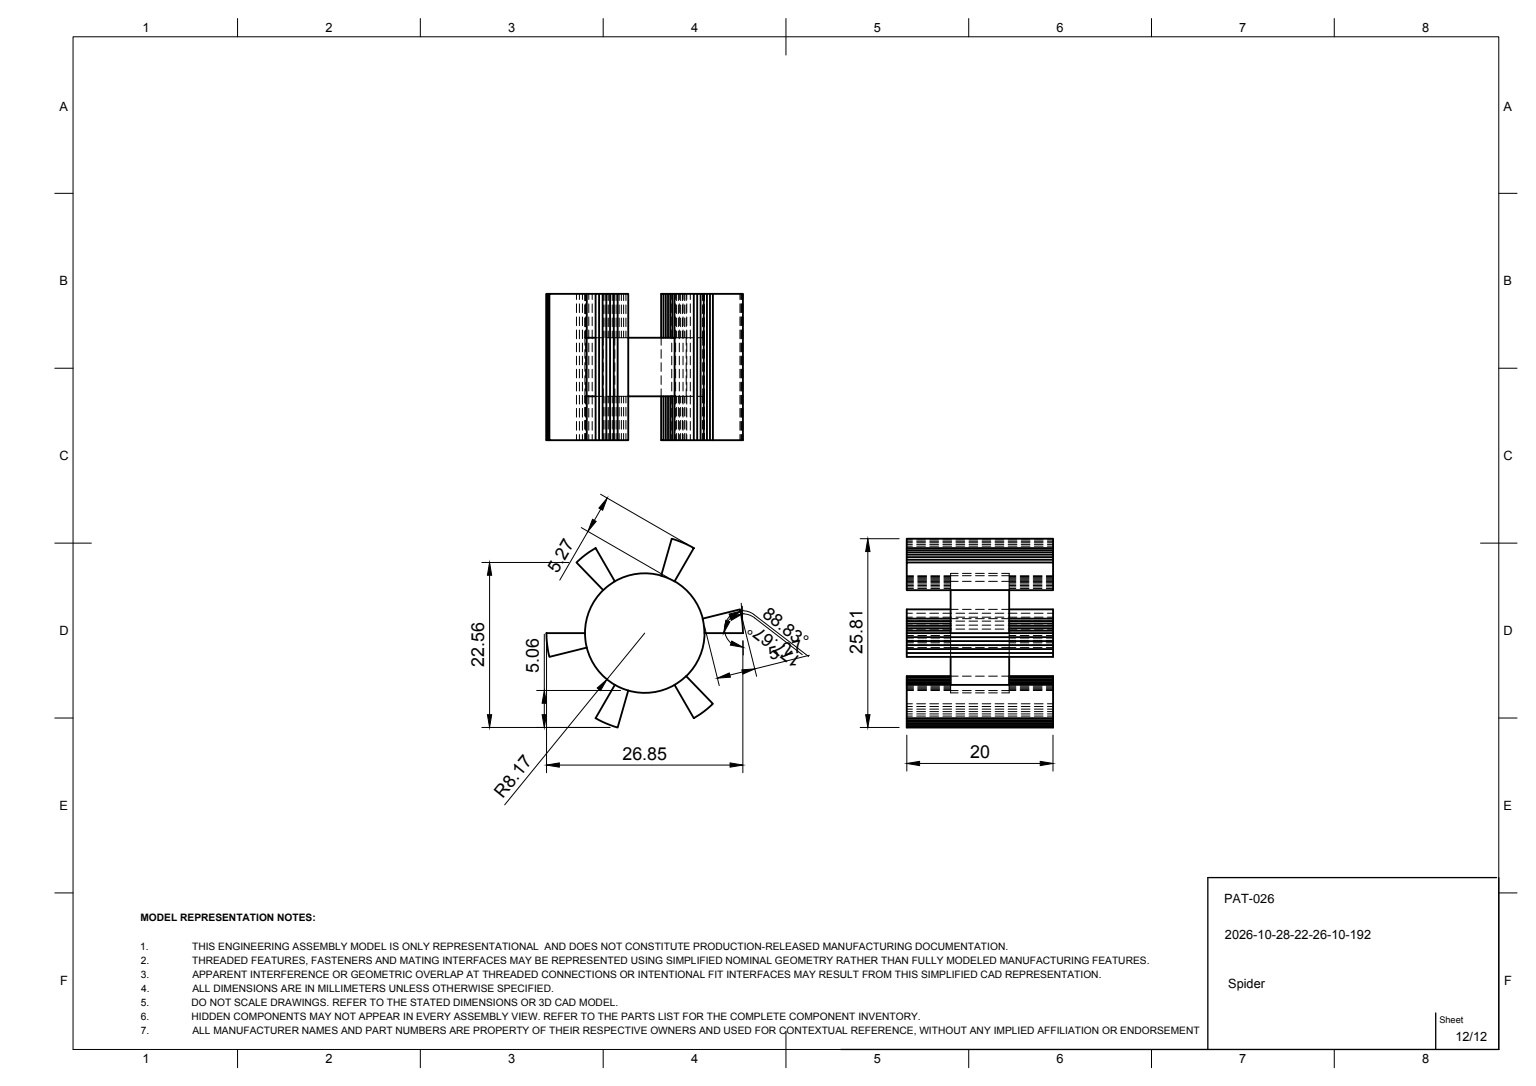
ISO-10303-21;
HEADER;
/* Generated by software containing ST-Developer
 * from STEP Tools, Inc. (www.steptools.com) 
 */

FILE_DESCRIPTION(
/* description */ ('PAT-026'),
/* implementation_level */ '2;1');

FILE_NAME(
/* name */ 'Spider.step',
/* time_stamp */ '2026-10-28T22:25:58-07:00',
/* author */ (''),
/* organization */ (''),
/* preprocessor_version */ 'ST-DEVELOPER v20.2',
/* originating_system */ 'Autodesk Translation Framework v15.17.0.0',
/* authorisation */ '');

FILE_SCHEMA (('AUTOMOTIVE_DESIGN { 1 0 10303 214 3 1 1 }'));
ENDSEC;

DATA;
#10=MECHANICAL_DESIGN_GEOMETRIC_PRESENTATION_REPRESENTATION('',(#150),#12343);
#128=SHAPE_REPRESENTATION_RELATIONSHIP('SRR','None',#12406,#139);
#139=ADVANCED_BREP_SHAPE_REPRESENTATION('',(#159),#12341);
#150=STYLED_ITEM('',(#12526),#159);
#159=MANIFOLD_SOLID_BREP('Body1',#7358);
#410=PLANE('',#7854);
#411=PLANE('',#7873);
#412=PLANE('',#7874);
#413=PLANE('',#7875);
#414=PLANE('',#7876);
#415=PLANE('',#7877);
#416=PLANE('',#7878);
#417=PLANE('',#7879);
#418=PLANE('',#7880);
#419=PLANE('',#7881);
#420=PLANE('',#7882);
#421=PLANE('',#7883);
#422=PLANE('',#7884);
#423=PLANE('',#7885);
#424=PLANE('',#7886);
#425=PLANE('',#7887);
#426=PLANE('',#7888);
#427=PLANE('',#7889);
#428=PLANE('',#7890);
#429=PLANE('',#7891);
#430=PLANE('',#7892);
#431=PLANE('',#7893);
#432=PLANE('',#7894);
#433=PLANE('',#7895);
#434=PLANE('',#7896);
#435=PLANE('',#7897);
#436=PLANE('',#7898);
#437=PLANE('',#7899);
#438=PLANE('',#7900);
#439=PLANE('',#7901);
#440=PLANE('',#7902);
#441=PLANE('',#7903);
#442=PLANE('',#7904);
#443=PLANE('',#7905);
#444=PLANE('',#7906);
#445=PLANE('',#7907);
#446=PLANE('',#7908);
#447=PLANE('',#7909);
#448=PLANE('',#7910);
#449=PLANE('',#7911);
#450=PLANE('',#7912);
#451=PLANE('',#7913);
#452=PLANE('',#7914);
#453=PLANE('',#7915);
#454=PLANE('',#7916);
#455=PLANE('',#7917);
#456=PLANE('',#7918);
#457=PLANE('',#7919);
#458=PLANE('',#7920);
#459=PLANE('',#7921);
#460=PLANE('',#7922);
#461=PLANE('',#7923);
#462=PLANE('',#7924);
#463=PLANE('',#7925);
#464=PLANE('',#7926);
#465=PLANE('',#7927);
#466=PLANE('',#7928);
#467=PLANE('',#7929);
#468=PLANE('',#7930);
#469=PLANE('',#7931);
#470=PLANE('',#7932);
#471=PLANE('',#7933);
#472=PLANE('',#7934);
#473=PLANE('',#7935);
#474=PLANE('',#7936);
#475=PLANE('',#7937);
#476=PLANE('',#7938);
#477=PLANE('',#7939);
#478=PLANE('',#7940);
#479=PLANE('',#7941);
#480=PLANE('',#7942);
#481=PLANE('',#7943);
#482=PLANE('',#7944);
#483=PLANE('',#7945);
#484=PLANE('',#7946);
#485=PLANE('',#7947);
#486=PLANE('',#7948);
#487=PLANE('',#7949);
#488=PLANE('',#7950);
#489=PLANE('',#7951);
#490=PLANE('',#7952);
#491=PLANE('',#7953);
#492=PLANE('',#7954);
#493=PLANE('',#7955);
#494=PLANE('',#7956);
#495=PLANE('',#7957);
#496=PLANE('',#7958);
#497=PLANE('',#7959);
#498=PLANE('',#7960);
#499=PLANE('',#7961);
#500=PLANE('',#7962);
#501=PLANE('',#7963);
#502=PLANE('',#7964);
#503=PLANE('',#7965);
#504=PLANE('',#7966);
#505=PLANE('',#7967);
#506=PLANE('',#7968);
#507=PLANE('',#7969);
#508=PLANE('',#7970);
#509=PLANE('',#7971);
#510=PLANE('',#7972);
#511=PLANE('',#7973);
#512=PLANE('',#7974);
#513=PLANE('',#7975);
#514=PLANE('',#7976);
#515=PLANE('',#7977);
#516=PLANE('',#7978);
#517=PLANE('',#7979);
#518=PLANE('',#7980);
#519=PLANE('',#7981);
#520=PLANE('',#7982);
#521=PLANE('',#7983);
#522=PLANE('',#7984);
#523=PLANE('',#7985);
#524=PLANE('',#7986);
#525=PLANE('',#7987);
#526=PLANE('',#7988);
#527=PLANE('',#7989);
#528=PLANE('',#7990);
#529=PLANE('',#7991);
#530=PLANE('',#7992);
#531=PLANE('',#7993);
#532=PLANE('',#7994);
#533=PLANE('',#7995);
#534=PLANE('',#7996);
#535=PLANE('',#7997);
#536=PLANE('',#7998);
#537=PLANE('',#7999);
#538=PLANE('',#8000);
#539=PLANE('',#8001);
#540=PLANE('',#8002);
#541=PLANE('',#8003);
#542=PLANE('',#8004);
#543=PLANE('',#8005);
#804=FACE_OUTER_BOUND('',#1239,.T.);
#805=FACE_OUTER_BOUND('',#1240,.T.);
#806=FACE_OUTER_BOUND('',#1241,.T.);
#807=FACE_OUTER_BOUND('',#1242,.T.);
#808=FACE_OUTER_BOUND('',#1243,.T.);
#809=FACE_OUTER_BOUND('',#1244,.T.);
#810=FACE_OUTER_BOUND('',#1245,.T.);
#811=FACE_OUTER_BOUND('',#1246,.T.);
#812=FACE_OUTER_BOUND('',#1247,.T.);
#813=FACE_OUTER_BOUND('',#1248,.T.);
#814=FACE_OUTER_BOUND('',#1249,.T.);
#815=FACE_OUTER_BOUND('',#1250,.T.);
#816=FACE_OUTER_BOUND('',#1251,.T.);
#817=FACE_OUTER_BOUND('',#1252,.T.);
#818=FACE_OUTER_BOUND('',#1253,.T.);
#819=FACE_OUTER_BOUND('',#1254,.T.);
#820=FACE_OUTER_BOUND('',#1255,.T.);
#821=FACE_OUTER_BOUND('',#1256,.T.);
#822=FACE_OUTER_BOUND('',#1257,.T.);
#823=FACE_OUTER_BOUND('',#1258,.T.);
#824=FACE_OUTER_BOUND('',#1259,.T.);
#825=FACE_OUTER_BOUND('',#1260,.T.);
#826=FACE_OUTER_BOUND('',#1261,.T.);
#827=FACE_OUTER_BOUND('',#1262,.T.);
#828=FACE_OUTER_BOUND('',#1263,.T.);
#829=FACE_OUTER_BOUND('',#1264,.T.);
#830=FACE_OUTER_BOUND('',#1265,.T.);
#831=FACE_OUTER_BOUND('',#1266,.T.);
#832=FACE_OUTER_BOUND('',#1267,.T.);
#833=FACE_OUTER_BOUND('',#1268,.T.);
#834=FACE_OUTER_BOUND('',#1269,.T.);
#835=FACE_OUTER_BOUND('',#1270,.T.);
#836=FACE_OUTER_BOUND('',#1271,.T.);
#837=FACE_OUTER_BOUND('',#1272,.T.);
#838=FACE_OUTER_BOUND('',#1273,.T.);
#839=FACE_OUTER_BOUND('',#1274,.T.);
#840=FACE_OUTER_BOUND('',#1275,.T.);
#841=FACE_OUTER_BOUND('',#1276,.T.);
#842=FACE_OUTER_BOUND('',#1277,.T.);
#843=FACE_OUTER_BOUND('',#1278,.T.);
#844=FACE_OUTER_BOUND('',#1279,.T.);
#845=FACE_OUTER_BOUND('',#1280,.T.);
#846=FACE_OUTER_BOUND('',#1281,.T.);
#847=FACE_OUTER_BOUND('',#1282,.T.);
#848=FACE_OUTER_BOUND('',#1283,.T.);
#849=FACE_OUTER_BOUND('',#1284,.T.);
#850=FACE_OUTER_BOUND('',#1285,.T.);
#851=FACE_OUTER_BOUND('',#1286,.T.);
#852=FACE_OUTER_BOUND('',#1287,.T.);
#853=FACE_OUTER_BOUND('',#1288,.T.);
#854=FACE_OUTER_BOUND('',#1289,.T.);
#855=FACE_OUTER_BOUND('',#1290,.T.);
#856=FACE_OUTER_BOUND('',#1291,.T.);
#857=FACE_OUTER_BOUND('',#1292,.T.);
#858=FACE_OUTER_BOUND('',#1293,.T.);
#859=FACE_OUTER_BOUND('',#1294,.T.);
#860=FACE_OUTER_BOUND('',#1295,.T.);
#861=FACE_OUTER_BOUND('',#1296,.T.);
#862=FACE_OUTER_BOUND('',#1297,.T.);
#863=FACE_OUTER_BOUND('',#1298,.T.);
#864=FACE_OUTER_BOUND('',#1299,.T.);
#865=FACE_OUTER_BOUND('',#1300,.T.);
#866=FACE_OUTER_BOUND('',#1301,.T.);
#867=FACE_OUTER_BOUND('',#1302,.T.);
#868=FACE_OUTER_BOUND('',#1303,.T.);
#869=FACE_OUTER_BOUND('',#1304,.T.);
#870=FACE_OUTER_BOUND('',#1305,.T.);
#871=FACE_OUTER_BOUND('',#1306,.T.);
#872=FACE_OUTER_BOUND('',#1307,.T.);
#873=FACE_OUTER_BOUND('',#1308,.T.);
#874=FACE_OUTER_BOUND('',#1309,.T.);
#875=FACE_OUTER_BOUND('',#1310,.T.);
#876=FACE_OUTER_BOUND('',#1311,.T.);
#877=FACE_OUTER_BOUND('',#1312,.T.);
#878=FACE_OUTER_BOUND('',#1313,.T.);
#879=FACE_OUTER_BOUND('',#1314,.T.);
#880=FACE_OUTER_BOUND('',#1315,.T.);
#881=FACE_OUTER_BOUND('',#1316,.T.);
#882=FACE_OUTER_BOUND('',#1317,.T.);
#883=FACE_OUTER_BOUND('',#1318,.T.);
#884=FACE_OUTER_BOUND('',#1319,.T.);
#885=FACE_OUTER_BOUND('',#1320,.T.);
#886=FACE_OUTER_BOUND('',#1321,.T.);
#887=FACE_OUTER_BOUND('',#1322,.T.);
#888=FACE_OUTER_BOUND('',#1323,.T.);
#889=FACE_OUTER_BOUND('',#1324,.T.);
#890=FACE_OUTER_BOUND('',#1325,.T.);
#891=FACE_OUTER_BOUND('',#1326,.T.);
#892=FACE_OUTER_BOUND('',#1327,.T.);
#893=FACE_OUTER_BOUND('',#1328,.T.);
#894=FACE_OUTER_BOUND('',#1329,.T.);
#895=FACE_OUTER_BOUND('',#1330,.T.);
#896=FACE_OUTER_BOUND('',#1331,.T.);
#897=FACE_OUTER_BOUND('',#1332,.T.);
#898=FACE_OUTER_BOUND('',#1333,.T.);
#899=FACE_OUTER_BOUND('',#1334,.T.);
#900=FACE_OUTER_BOUND('',#1335,.T.);
#901=FACE_OUTER_BOUND('',#1336,.T.);
#902=FACE_OUTER_BOUND('',#1337,.T.);
#903=FACE_OUTER_BOUND('',#1338,.T.);
#904=FACE_OUTER_BOUND('',#1339,.T.);
#905=FACE_OUTER_BOUND('',#1340,.T.);
#906=FACE_OUTER_BOUND('',#1341,.T.);
#907=FACE_OUTER_BOUND('',#1342,.T.);
#908=FACE_OUTER_BOUND('',#1343,.T.);
#909=FACE_OUTER_BOUND('',#1344,.T.);
#910=FACE_OUTER_BOUND('',#1345,.T.);
#911=FACE_OUTER_BOUND('',#1346,.T.);
#912=FACE_OUTER_BOUND('',#1347,.T.);
#913=FACE_OUTER_BOUND('',#1348,.T.);
#914=FACE_OUTER_BOUND('',#1349,.T.);
#915=FACE_OUTER_BOUND('',#1350,.T.);
#916=FACE_OUTER_BOUND('',#1351,.T.);
#917=FACE_OUTER_BOUND('',#1352,.T.);
#918=FACE_OUTER_BOUND('',#1353,.T.);
#919=FACE_OUTER_BOUND('',#1354,.T.);
#920=FACE_OUTER_BOUND('',#1355,.T.);
#921=FACE_OUTER_BOUND('',#1356,.T.);
#922=FACE_OUTER_BOUND('',#1357,.T.);
#923=FACE_OUTER_BOUND('',#1358,.T.);
#924=FACE_OUTER_BOUND('',#1359,.T.);
#925=FACE_OUTER_BOUND('',#1360,.T.);
#926=FACE_OUTER_BOUND('',#1361,.T.);
#927=FACE_OUTER_BOUND('',#1362,.T.);
#928=FACE_OUTER_BOUND('',#1363,.T.);
#929=FACE_OUTER_BOUND('',#1364,.T.);
#930=FACE_OUTER_BOUND('',#1365,.T.);
#931=FACE_OUTER_BOUND('',#1366,.T.);
#932=FACE_OUTER_BOUND('',#1367,.T.);
#933=FACE_OUTER_BOUND('',#1368,.T.);
#934=FACE_OUTER_BOUND('',#1369,.T.);
#935=FACE_OUTER_BOUND('',#1370,.T.);
#936=FACE_OUTER_BOUND('',#1371,.T.);
#937=FACE_OUTER_BOUND('',#1372,.T.);
#938=FACE_OUTER_BOUND('',#1373,.T.);
#939=FACE_OUTER_BOUND('',#1374,.T.);
#940=FACE_OUTER_BOUND('',#1375,.T.);
#941=FACE_OUTER_BOUND('',#1376,.T.);
#942=FACE_OUTER_BOUND('',#1377,.T.);
#943=FACE_OUTER_BOUND('',#1378,.T.);
#1239=EDGE_LOOP('',(#6033,#6034,#6035,#6036,#6037,#6038,#6039,#6040,#6041,
#6042,#6043,#6044,#6045,#6046,#6047,#6048,#6049,#6050,#6051,#6052,#6053,
#6054,#6055,#6056,#6057,#6058,#6059,#6060,#6061,#6062,#6063,#6064,#6065,
#6066,#6067,#6068,#6069,#6070,#6071,#6072,#6073,#6074,#6075,#6076,#6077,
#6078,#6079,#6080,#6081,#6082,#6083,#6084,#6085,#6086));
#1240=EDGE_LOOP('',(#6087,#6088,#6089,#6090));
#1241=EDGE_LOOP('',(#6091,#6092,#6093,#6094));
#1242=EDGE_LOOP('',(#6095,#6096,#6097,#6098));
#1243=EDGE_LOOP('',(#6099,#6100,#6101,#6102));
#1244=EDGE_LOOP('',(#6103,#6104,#6105,#6106));
#1245=EDGE_LOOP('',(#6107,#6108,#6109,#6110));
#1246=EDGE_LOOP('',(#6111,#6112,#6113,#6114,#6115,#6116,#6117,#6118,#6119,
#6120,#6121,#6122,#6123,#6124,#6125,#6126,#6127,#6128,#6129,#6130,#6131,
#6132,#6133,#6134,#6135,#6136,#6137,#6138,#6139,#6140,#6141,#6142,#6143,
#6144,#6145,#6146,#6147,#6148,#6149,#6150,#6151,#6152,#6153,#6154,#6155,
#6156,#6157,#6158,#6159,#6160,#6161,#6162,#6163,#6164));
#1247=EDGE_LOOP('',(#6165,#6166,#6167,#6168,#6169,#6170,#6171,#6172));
#1248=EDGE_LOOP('',(#6173,#6174,#6175,#6176));
#1249=EDGE_LOOP('',(#6177,#6178,#6179,#6180));
#1250=EDGE_LOOP('',(#6181,#6182,#6183,#6184));
#1251=EDGE_LOOP('',(#6185,#6186,#6187,#6188));
#1252=EDGE_LOOP('',(#6189,#6190,#6191,#6192));
#1253=EDGE_LOOP('',(#6193,#6194,#6195,#6196));
#1254=EDGE_LOOP('',(#6197,#6198,#6199,#6200));
#1255=EDGE_LOOP('',(#6201,#6202,#6203,#6204,#6205,#6206,#6207,#6208,#6209,
#6210,#6211,#6212,#6213,#6214));
#1256=EDGE_LOOP('',(#6215,#6216,#6217,#6218));
#1257=EDGE_LOOP('',(#6219,#6220,#6221,#6222));
#1258=EDGE_LOOP('',(#6223,#6224,#6225,#6226));
#1259=EDGE_LOOP('',(#6227,#6228,#6229,#6230));
#1260=EDGE_LOOP('',(#6231,#6232,#6233,#6234));
#1261=EDGE_LOOP('',(#6235,#6236,#6237,#6238));
#1262=EDGE_LOOP('',(#6239,#6240,#6241,#6242));
#1263=EDGE_LOOP('',(#6243,#6244,#6245,#6246));
#1264=EDGE_LOOP('',(#6247,#6248,#6249,#6250));
#1265=EDGE_LOOP('',(#6251,#6252,#6253,#6254));
#1266=EDGE_LOOP('',(#6255,#6256,#6257,#6258));
#1267=EDGE_LOOP('',(#6259,#6260,#6261,#6262,#6263,#6264,#6265,#6266));
#1268=EDGE_LOOP('',(#6267,#6268,#6269,#6270,#6271,#6272,#6273,#6274,#6275,
#6276,#6277,#6278,#6279,#6280));
#1269=EDGE_LOOP('',(#6281,#6282,#6283,#6284,#6285,#6286,#6287,#6288));
#1270=EDGE_LOOP('',(#6289,#6290,#6291,#6292));
#1271=EDGE_LOOP('',(#6293,#6294,#6295,#6296));
#1272=EDGE_LOOP('',(#6297,#6298,#6299,#6300));
#1273=EDGE_LOOP('',(#6301,#6302,#6303,#6304));
#1274=EDGE_LOOP('',(#6305,#6306,#6307,#6308));
#1275=EDGE_LOOP('',(#6309,#6310,#6311,#6312));
#1276=EDGE_LOOP('',(#6313,#6314,#6315,#6316));
#1277=EDGE_LOOP('',(#6317,#6318,#6319,#6320,#6321,#6322,#6323,#6324,#6325,
#6326,#6327,#6328,#6329,#6330));
#1278=EDGE_LOOP('',(#6331,#6332,#6333,#6334));
#1279=EDGE_LOOP('',(#6335,#6336,#6337,#6338));
#1280=EDGE_LOOP('',(#6339,#6340,#6341,#6342));
#1281=EDGE_LOOP('',(#6343,#6344,#6345,#6346));
#1282=EDGE_LOOP('',(#6347,#6348,#6349,#6350));
#1283=EDGE_LOOP('',(#6351,#6352,#6353,#6354));
#1284=EDGE_LOOP('',(#6355,#6356,#6357,#6358));
#1285=EDGE_LOOP('',(#6359,#6360,#6361,#6362));
#1286=EDGE_LOOP('',(#6363,#6364,#6365,#6366));
#1287=EDGE_LOOP('',(#6367,#6368,#6369,#6370));
#1288=EDGE_LOOP('',(#6371,#6372,#6373,#6374));
#1289=EDGE_LOOP('',(#6375,#6376,#6377,#6378,#6379,#6380,#6381,#6382));
#1290=EDGE_LOOP('',(#6383,#6384,#6385,#6386,#6387,#6388,#6389,#6390,#6391,
#6392,#6393,#6394,#6395,#6396));
#1291=EDGE_LOOP('',(#6397,#6398,#6399,#6400,#6401,#6402,#6403,#6404));
#1292=EDGE_LOOP('',(#6405,#6406,#6407,#6408));
#1293=EDGE_LOOP('',(#6409,#6410,#6411,#6412));
#1294=EDGE_LOOP('',(#6413,#6414,#6415,#6416));
#1295=EDGE_LOOP('',(#6417,#6418,#6419,#6420));
#1296=EDGE_LOOP('',(#6421,#6422,#6423,#6424));
#1297=EDGE_LOOP('',(#6425,#6426,#6427,#6428));
#1298=EDGE_LOOP('',(#6429,#6430,#6431,#6432));
#1299=EDGE_LOOP('',(#6433,#6434,#6435,#6436,#6437,#6438,#6439,#6440,#6441,
#6442,#6443,#6444,#6445,#6446));
#1300=EDGE_LOOP('',(#6447,#6448,#6449,#6450));
#1301=EDGE_LOOP('',(#6451,#6452,#6453,#6454));
#1302=EDGE_LOOP('',(#6455,#6456,#6457,#6458));
#1303=EDGE_LOOP('',(#6459,#6460,#6461,#6462));
#1304=EDGE_LOOP('',(#6463,#6464,#6465,#6466));
#1305=EDGE_LOOP('',(#6467,#6468,#6469,#6470));
#1306=EDGE_LOOP('',(#6471,#6472,#6473,#6474));
#1307=EDGE_LOOP('',(#6475,#6476,#6477,#6478));
#1308=EDGE_LOOP('',(#6479,#6480,#6481,#6482));
#1309=EDGE_LOOP('',(#6483,#6484,#6485,#6486));
#1310=EDGE_LOOP('',(#6487,#6488,#6489,#6490));
#1311=EDGE_LOOP('',(#6491,#6492,#6493,#6494,#6495,#6496,#6497,#6498));
#1312=EDGE_LOOP('',(#6499,#6500,#6501,#6502,#6503,#6504,#6505,#6506,#6507,
#6508,#6509,#6510,#6511,#6512));
#1313=EDGE_LOOP('',(#6513,#6514,#6515,#6516,#6517,#6518,#6519,#6520));
#1314=EDGE_LOOP('',(#6521,#6522,#6523,#6524));
#1315=EDGE_LOOP('',(#6525,#6526,#6527,#6528));
#1316=EDGE_LOOP('',(#6529,#6530,#6531,#6532));
#1317=EDGE_LOOP('',(#6533,#6534,#6535,#6536));
#1318=EDGE_LOOP('',(#6537,#6538,#6539,#6540));
#1319=EDGE_LOOP('',(#6541,#6542,#6543,#6544));
#1320=EDGE_LOOP('',(#6545,#6546,#6547,#6548));
#1321=EDGE_LOOP('',(#6549,#6550,#6551,#6552,#6553,#6554,#6555,#6556,#6557,
#6558,#6559,#6560,#6561,#6562));
#1322=EDGE_LOOP('',(#6563,#6564,#6565,#6566));
#1323=EDGE_LOOP('',(#6567,#6568,#6569,#6570));
#1324=EDGE_LOOP('',(#6571,#6572,#6573,#6574));
#1325=EDGE_LOOP('',(#6575,#6576,#6577,#6578));
#1326=EDGE_LOOP('',(#6579,#6580,#6581,#6582));
#1327=EDGE_LOOP('',(#6583,#6584,#6585,#6586));
#1328=EDGE_LOOP('',(#6587,#6588,#6589,#6590));
#1329=EDGE_LOOP('',(#6591,#6592,#6593,#6594));
#1330=EDGE_LOOP('',(#6595,#6596,#6597,#6598));
#1331=EDGE_LOOP('',(#6599,#6600,#6601,#6602));
#1332=EDGE_LOOP('',(#6603,#6604,#6605,#6606));
#1333=EDGE_LOOP('',(#6607,#6608,#6609,#6610,#6611,#6612,#6613,#6614));
#1334=EDGE_LOOP('',(#6615,#6616,#6617,#6618,#6619,#6620,#6621,#6622,#6623,
#6624,#6625,#6626,#6627,#6628));
#1335=EDGE_LOOP('',(#6629,#6630,#6631,#6632,#6633,#6634,#6635,#6636));
#1336=EDGE_LOOP('',(#6637,#6638,#6639,#6640));
#1337=EDGE_LOOP('',(#6641,#6642,#6643,#6644));
#1338=EDGE_LOOP('',(#6645,#6646,#6647,#6648));
#1339=EDGE_LOOP('',(#6649,#6650,#6651,#6652));
#1340=EDGE_LOOP('',(#6653,#6654,#6655,#6656));
#1341=EDGE_LOOP('',(#6657,#6658,#6659,#6660));
#1342=EDGE_LOOP('',(#6661,#6662,#6663,#6664));
#1343=EDGE_LOOP('',(#6665,#6666,#6667,#6668,#6669,#6670,#6671,#6672,#6673,
#6674,#6675,#6676,#6677,#6678));
#1344=EDGE_LOOP('',(#6679,#6680,#6681,#6682));
#1345=EDGE_LOOP('',(#6683,#6684,#6685,#6686));
#1346=EDGE_LOOP('',(#6687,#6688,#6689,#6690));
#1347=EDGE_LOOP('',(#6691,#6692,#6693,#6694));
#1348=EDGE_LOOP('',(#6695,#6696,#6697,#6698));
#1349=EDGE_LOOP('',(#6699,#6700,#6701,#6702));
#1350=EDGE_LOOP('',(#6703,#6704,#6705,#6706));
#1351=EDGE_LOOP('',(#6707,#6708,#6709,#6710));
#1352=EDGE_LOOP('',(#6711,#6712,#6713,#6714));
#1353=EDGE_LOOP('',(#6715,#6716,#6717,#6718));
#1354=EDGE_LOOP('',(#6719,#6720,#6721,#6722));
#1355=EDGE_LOOP('',(#6723,#6724,#6725,#6726,#6727,#6728,#6729,#6730));
#1356=EDGE_LOOP('',(#6731,#6732,#6733,#6734,#6735,#6736,#6737,#6738,#6739,
#6740,#6741,#6742,#6743,#6744));
#1357=EDGE_LOOP('',(#6745,#6746,#6747,#6748,#6749,#6750,#6751,#6752));
#1358=EDGE_LOOP('',(#6753,#6754,#6755,#6756));
#1359=EDGE_LOOP('',(#6757,#6758,#6759,#6760));
#1360=EDGE_LOOP('',(#6761,#6762,#6763,#6764));
#1361=EDGE_LOOP('',(#6765,#6766,#6767,#6768));
#1362=EDGE_LOOP('',(#6769,#6770,#6771,#6772));
#1363=EDGE_LOOP('',(#6773,#6774,#6775,#6776));
#1364=EDGE_LOOP('',(#6777,#6778,#6779,#6780));
#1365=EDGE_LOOP('',(#6781,#6782,#6783,#6784,#6785,#6786,#6787,#6788,#6789,
#6790,#6791,#6792,#6793,#6794));
#1366=EDGE_LOOP('',(#6795,#6796,#6797,#6798));
#1367=EDGE_LOOP('',(#6799,#6800,#6801,#6802));
#1368=EDGE_LOOP('',(#6803,#6804,#6805,#6806));
#1369=EDGE_LOOP('',(#6807,#6808,#6809,#6810));
#1370=EDGE_LOOP('',(#6811,#6812,#6813,#6814));
#1371=EDGE_LOOP('',(#6815,#6816,#6817,#6818));
#1372=EDGE_LOOP('',(#6819,#6820,#6821,#6822));
#1373=EDGE_LOOP('',(#6823,#6824,#6825,#6826));
#1374=EDGE_LOOP('',(#6827,#6828,#6829,#6830));
#1375=EDGE_LOOP('',(#6831,#6832,#6833,#6834));
#1376=EDGE_LOOP('',(#6835,#6836,#6837,#6838));
#1377=EDGE_LOOP('',(#6839,#6840,#6841,#6842,#6843,#6844,#6845,#6846));
#1378=EDGE_LOOP('',(#6847,#6848,#6849,#6850,#6851,#6852,#6853,#6854,#6855,
#6856,#6857,#6858,#6859,#6860));
#1841=LINE('',#11414,#2713);
#1842=LINE('',#11416,#2714);
#1843=LINE('',#11418,#2715);
#1844=LINE('',#11420,#2716);
#1845=LINE('',#11422,#2717);
#1846=LINE('',#11424,#2718);
#1847=LINE('',#11426,#2719);
#1848=LINE('',#11428,#2720);
#1849=LINE('',#11432,#2721);
#1850=LINE('',#11434,#2722);
#1851=LINE('',#11436,#2723);
#1852=LINE('',#11438,#2724);
#1853=LINE('',#11440,#2725);
#1854=LINE('',#11442,#2726);
#1855=LINE('',#11444,#2727);
#1856=LINE('',#11446,#2728);
#1857=LINE('',#11450,#2729);
#1858=LINE('',#11452,#2730);
#1859=LINE('',#11454,#2731);
#1860=LINE('',#11456,#2732);
#1861=LINE('',#11458,#2733);
#1862=LINE('',#11460,#2734);
#1863=LINE('',#11462,#2735);
#1864=LINE('',#11464,#2736);
#1865=LINE('',#11468,#2737);
#1866=LINE('',#11470,#2738);
#1867=LINE('',#11472,#2739);
#1868=LINE('',#11474,#2740);
#1869=LINE('',#11476,#2741);
#1870=LINE('',#11478,#2742);
#1871=LINE('',#11480,#2743);
#1872=LINE('',#11482,#2744);
#1873=LINE('',#11486,#2745);
#1874=LINE('',#11488,#2746);
#1875=LINE('',#11490,#2747);
#1876=LINE('',#11492,#2748);
#1877=LINE('',#11494,#2749);
#1878=LINE('',#11496,#2750);
#1879=LINE('',#11498,#2751);
#1880=LINE('',#11500,#2752);
#1881=LINE('',#11504,#2753);
#1882=LINE('',#11506,#2754);
#1883=LINE('',#11508,#2755);
#1884=LINE('',#11510,#2756);
#1885=LINE('',#11512,#2757);
#1886=LINE('',#11514,#2758);
#1887=LINE('',#11516,#2759);
#1888=LINE('',#11518,#2760);
#1889=LINE('',#11522,#2761);
#1890=LINE('',#11525,#2762);
#1891=LINE('',#11528,#2763);
#1892=LINE('',#11531,#2764);
#1893=LINE('',#11534,#2765);
#1894=LINE('',#11537,#2766);
#1895=LINE('',#11540,#2767);
#1896=LINE('',#11542,#2768);
#1897=LINE('',#11546,#2769);
#1898=LINE('',#11548,#2770);
#1899=LINE('',#11552,#2771);
#1900=LINE('',#11554,#2772);
#1901=LINE('',#11558,#2773);
#1902=LINE('',#11560,#2774);
#1903=LINE('',#11562,#2775);
#1904=LINE('',#11564,#2776);
#1905=LINE('',#11566,#2777);
#1906=LINE('',#11568,#2778);
#1907=LINE('',#11570,#2779);
#1908=LINE('',#11572,#2780);
#1909=LINE('',#11573,#2781);
#1910=LINE('',#11575,#2782);
#1911=LINE('',#11577,#2783);
#1912=LINE('',#11579,#2784);
#1913=LINE('',#11581,#2785);
#1914=LINE('',#11583,#2786);
#1915=LINE('',#11585,#2787);
#1916=LINE('',#11587,#2788);
#1917=LINE('',#11588,#2789);
#1918=LINE('',#11590,#2790);
#1919=LINE('',#11592,#2791);
#1920=LINE('',#11594,#2792);
#1921=LINE('',#11596,#2793);
#1922=LINE('',#11598,#2794);
#1923=LINE('',#11600,#2795);
#1924=LINE('',#11602,#2796);
#1925=LINE('',#11603,#2797);
#1926=LINE('',#11605,#2798);
#1927=LINE('',#11607,#2799);
#1928=LINE('',#11609,#2800);
#1929=LINE('',#11611,#2801);
#1930=LINE('',#11613,#2802);
#1931=LINE('',#11615,#2803);
#1932=LINE('',#11617,#2804);
#1933=LINE('',#11618,#2805);
#1934=LINE('',#11620,#2806);
#1935=LINE('',#11622,#2807);
#1936=LINE('',#11624,#2808);
#1937=LINE('',#11626,#2809);
#1938=LINE('',#11628,#2810);
#1939=LINE('',#11630,#2811);
#1940=LINE('',#11632,#2812);
#1941=LINE('',#11633,#2813);
#1942=LINE('',#11635,#2814);
#1943=LINE('',#11637,#2815);
#1944=LINE('',#11639,#2816);
#1945=LINE('',#11641,#2817);
#1946=LINE('',#11643,#2818);
#1947=LINE('',#11645,#2819);
#1948=LINE('',#11646,#2820);
#1949=LINE('',#11649,#2821);
#1950=LINE('',#11651,#2822);
#1951=LINE('',#11653,#2823);
#1952=LINE('',#11655,#2824);
#1953=LINE('',#11656,#2825);
#1954=LINE('',#11659,#2826);
#1955=LINE('',#11660,#2827);
#1956=LINE('',#11663,#2828);
#1957=LINE('',#11664,#2829);
#1958=LINE('',#11667,#2830);
#1959=LINE('',#11668,#2831);
#1960=LINE('',#11671,#2832);
#1961=LINE('',#11672,#2833);
#1962=LINE('',#11675,#2834);
#1963=LINE('',#11676,#2835);
#1964=LINE('',#11679,#2836);
#1965=LINE('',#11680,#2837);
#1966=LINE('',#11683,#2838);
#1967=LINE('',#11684,#2839);
#1968=LINE('',#11688,#2840);
#1969=LINE('',#11690,#2841);
#1970=LINE('',#11692,#2842);
#1971=LINE('',#11694,#2843);
#1972=LINE('',#11696,#2844);
#1973=LINE('',#11697,#2845);
#1974=LINE('',#11699,#2846);
#1975=LINE('',#11701,#2847);
#1976=LINE('',#11703,#2848);
#1977=LINE('',#11705,#2849);
#1978=LINE('',#11707,#2850);
#1979=LINE('',#11708,#2851);
#1980=LINE('',#11710,#2852);
#1981=LINE('',#11711,#2853);
#1982=LINE('',#11713,#2854);
#1983=LINE('',#11715,#2855);
#1984=LINE('',#11717,#2856);
#1985=LINE('',#11721,#2857);
#1986=LINE('',#11722,#2858);
#1987=LINE('',#11725,#2859);
#1988=LINE('',#11726,#2860);
#1989=LINE('',#11729,#2861);
#1990=LINE('',#11730,#2862);
#1991=LINE('',#11733,#2863);
#1992=LINE('',#11734,#2864);
#1993=LINE('',#11737,#2865);
#1994=LINE('',#11738,#2866);
#1995=LINE('',#11741,#2867);
#1996=LINE('',#11742,#2868);
#1997=LINE('',#11744,#2869);
#1998=LINE('',#11748,#2870);
#1999=LINE('',#11750,#2871);
#2000=LINE('',#11752,#2872);
#2001=LINE('',#11754,#2873);
#2002=LINE('',#11755,#2874);
#2003=LINE('',#11758,#2875);
#2004=LINE('',#11759,#2876);
#2005=LINE('',#11762,#2877);
#2006=LINE('',#11763,#2878);
#2007=LINE('',#11766,#2879);
#2008=LINE('',#11767,#2880);
#2009=LINE('',#11770,#2881);
#2010=LINE('',#11771,#2882);
#2011=LINE('',#11774,#2883);
#2012=LINE('',#11775,#2884);
#2013=LINE('',#11778,#2885);
#2014=LINE('',#11779,#2886);
#2015=LINE('',#11782,#2887);
#2016=LINE('',#11783,#2888);
#2017=LINE('',#11787,#2889);
#2018=LINE('',#11789,#2890);
#2019=LINE('',#11791,#2891);
#2020=LINE('',#11793,#2892);
#2021=LINE('',#11795,#2893);
#2022=LINE('',#11796,#2894);
#2023=LINE('',#11798,#2895);
#2024=LINE('',#11800,#2896);
#2025=LINE('',#11802,#2897);
#2026=LINE('',#11804,#2898);
#2027=LINE('',#11806,#2899);
#2028=LINE('',#11807,#2900);
#2029=LINE('',#11809,#2901);
#2030=LINE('',#11810,#2902);
#2031=LINE('',#11812,#2903);
#2032=LINE('',#11814,#2904);
#2033=LINE('',#11816,#2905);
#2034=LINE('',#11820,#2906);
#2035=LINE('',#11821,#2907);
#2036=LINE('',#11824,#2908);
#2037=LINE('',#11825,#2909);
#2038=LINE('',#11828,#2910);
#2039=LINE('',#11829,#2911);
#2040=LINE('',#11832,#2912);
#2041=LINE('',#11833,#2913);
#2042=LINE('',#11836,#2914);
#2043=LINE('',#11837,#2915);
#2044=LINE('',#11840,#2916);
#2045=LINE('',#11841,#2917);
#2046=LINE('',#11843,#2918);
#2047=LINE('',#11847,#2919);
#2048=LINE('',#11849,#2920);
#2049=LINE('',#11851,#2921);
#2050=LINE('',#11853,#2922);
#2051=LINE('',#11854,#2923);
#2052=LINE('',#11857,#2924);
#2053=LINE('',#11858,#2925);
#2054=LINE('',#11861,#2926);
#2055=LINE('',#11862,#2927);
#2056=LINE('',#11865,#2928);
#2057=LINE('',#11866,#2929);
#2058=LINE('',#11869,#2930);
#2059=LINE('',#11870,#2931);
#2060=LINE('',#11873,#2932);
#2061=LINE('',#11874,#2933);
#2062=LINE('',#11877,#2934);
#2063=LINE('',#11878,#2935);
#2064=LINE('',#11881,#2936);
#2065=LINE('',#11882,#2937);
#2066=LINE('',#11886,#2938);
#2067=LINE('',#11888,#2939);
#2068=LINE('',#11890,#2940);
#2069=LINE('',#11892,#2941);
#2070=LINE('',#11894,#2942);
#2071=LINE('',#11895,#2943);
#2072=LINE('',#11897,#2944);
#2073=LINE('',#11899,#2945);
#2074=LINE('',#11901,#2946);
#2075=LINE('',#11903,#2947);
#2076=LINE('',#11905,#2948);
#2077=LINE('',#11906,#2949);
#2078=LINE('',#11908,#2950);
#2079=LINE('',#11909,#2951);
#2080=LINE('',#11911,#2952);
#2081=LINE('',#11913,#2953);
#2082=LINE('',#11915,#2954);
#2083=LINE('',#11919,#2955);
#2084=LINE('',#11920,#2956);
#2085=LINE('',#11923,#2957);
#2086=LINE('',#11924,#2958);
#2087=LINE('',#11927,#2959);
#2088=LINE('',#11928,#2960);
#2089=LINE('',#11931,#2961);
#2090=LINE('',#11932,#2962);
#2091=LINE('',#11935,#2963);
#2092=LINE('',#11936,#2964);
#2093=LINE('',#11939,#2965);
#2094=LINE('',#11940,#2966);
#2095=LINE('',#11942,#2967);
#2096=LINE('',#11946,#2968);
#2097=LINE('',#11948,#2969);
#2098=LINE('',#11950,#2970);
#2099=LINE('',#11952,#2971);
#2100=LINE('',#11953,#2972);
#2101=LINE('',#11956,#2973);
#2102=LINE('',#11957,#2974);
#2103=LINE('',#11960,#2975);
#2104=LINE('',#11961,#2976);
#2105=LINE('',#11964,#2977);
#2106=LINE('',#11965,#2978);
#2107=LINE('',#11968,#2979);
#2108=LINE('',#11969,#2980);
#2109=LINE('',#11972,#2981);
#2110=LINE('',#11973,#2982);
#2111=LINE('',#11976,#2983);
#2112=LINE('',#11977,#2984);
#2113=LINE('',#11980,#2985);
#2114=LINE('',#11981,#2986);
#2115=LINE('',#11985,#2987);
#2116=LINE('',#11987,#2988);
#2117=LINE('',#11989,#2989);
#2118=LINE('',#11991,#2990);
#2119=LINE('',#11993,#2991);
#2120=LINE('',#11994,#2992);
#2121=LINE('',#11996,#2993);
#2122=LINE('',#11998,#2994);
#2123=LINE('',#12000,#2995);
#2124=LINE('',#12002,#2996);
#2125=LINE('',#12004,#2997);
#2126=LINE('',#12005,#2998);
#2127=LINE('',#12007,#2999);
#2128=LINE('',#12008,#3000);
#2129=LINE('',#12010,#3001);
#2130=LINE('',#12012,#3002);
#2131=LINE('',#12014,#3003);
#2132=LINE('',#12018,#3004);
#2133=LINE('',#12019,#3005);
#2134=LINE('',#12022,#3006);
#2135=LINE('',#12023,#3007);
#2136=LINE('',#12026,#3008);
#2137=LINE('',#12027,#3009);
#2138=LINE('',#12030,#3010);
#2139=LINE('',#12031,#3011);
#2140=LINE('',#12034,#3012);
#2141=LINE('',#12035,#3013);
#2142=LINE('',#12038,#3014);
#2143=LINE('',#12039,#3015);
#2144=LINE('',#12041,#3016);
#2145=LINE('',#12045,#3017);
#2146=LINE('',#12047,#3018);
#2147=LINE('',#12049,#3019);
#2148=LINE('',#12051,#3020);
#2149=LINE('',#12052,#3021);
#2150=LINE('',#12055,#3022);
#2151=LINE('',#12056,#3023);
#2152=LINE('',#12059,#3024);
#2153=LINE('',#12060,#3025);
#2154=LINE('',#12063,#3026);
#2155=LINE('',#12064,#3027);
#2156=LINE('',#12067,#3028);
#2157=LINE('',#12068,#3029);
#2158=LINE('',#12071,#3030);
#2159=LINE('',#12072,#3031);
#2160=LINE('',#12075,#3032);
#2161=LINE('',#12076,#3033);
#2162=LINE('',#12079,#3034);
#2163=LINE('',#12080,#3035);
#2164=LINE('',#12084,#3036);
#2165=LINE('',#12086,#3037);
#2166=LINE('',#12088,#3038);
#2167=LINE('',#12090,#3039);
#2168=LINE('',#12092,#3040);
#2169=LINE('',#12093,#3041);
#2170=LINE('',#12095,#3042);
#2171=LINE('',#12097,#3043);
#2172=LINE('',#12099,#3044);
#2173=LINE('',#12101,#3045);
#2174=LINE('',#12103,#3046);
#2175=LINE('',#12104,#3047);
#2176=LINE('',#12106,#3048);
#2177=LINE('',#12107,#3049);
#2178=LINE('',#12109,#3050);
#2179=LINE('',#12111,#3051);
#2180=LINE('',#12113,#3052);
#2181=LINE('',#12117,#3053);
#2182=LINE('',#12118,#3054);
#2183=LINE('',#12121,#3055);
#2184=LINE('',#12122,#3056);
#2185=LINE('',#12125,#3057);
#2186=LINE('',#12126,#3058);
#2187=LINE('',#12129,#3059);
#2188=LINE('',#12130,#3060);
#2189=LINE('',#12133,#3061);
#2190=LINE('',#12134,#3062);
#2191=LINE('',#12137,#3063);
#2192=LINE('',#12138,#3064);
#2193=LINE('',#12140,#3065);
#2194=LINE('',#12144,#3066);
#2195=LINE('',#12146,#3067);
#2196=LINE('',#12148,#3068);
#2197=LINE('',#12150,#3069);
#2198=LINE('',#12151,#3070);
#2199=LINE('',#12154,#3071);
#2200=LINE('',#12155,#3072);
#2201=LINE('',#12158,#3073);
#2202=LINE('',#12159,#3074);
#2203=LINE('',#12162,#3075);
#2204=LINE('',#12163,#3076);
#2205=LINE('',#12166,#3077);
#2206=LINE('',#12167,#3078);
#2207=LINE('',#12170,#3079);
#2208=LINE('',#12171,#3080);
#2209=LINE('',#12174,#3081);
#2210=LINE('',#12175,#3082);
#2211=LINE('',#12178,#3083);
#2212=LINE('',#12179,#3084);
#2213=LINE('',#12183,#3085);
#2214=LINE('',#12185,#3086);
#2215=LINE('',#12187,#3087);
#2216=LINE('',#12189,#3088);
#2217=LINE('',#12191,#3089);
#2218=LINE('',#12192,#3090);
#2219=LINE('',#12194,#3091);
#2220=LINE('',#12196,#3092);
#2221=LINE('',#12198,#3093);
#2222=LINE('',#12200,#3094);
#2223=LINE('',#12202,#3095);
#2224=LINE('',#12203,#3096);
#2225=LINE('',#12205,#3097);
#2226=LINE('',#12206,#3098);
#2227=LINE('',#12208,#3099);
#2228=LINE('',#12210,#3100);
#2229=LINE('',#12212,#3101);
#2230=LINE('',#12216,#3102);
#2231=LINE('',#12217,#3103);
#2232=LINE('',#12220,#3104);
#2233=LINE('',#12221,#3105);
#2234=LINE('',#12224,#3106);
#2235=LINE('',#12225,#3107);
#2236=LINE('',#12228,#3108);
#2237=LINE('',#12229,#3109);
#2238=LINE('',#12232,#3110);
#2239=LINE('',#12233,#3111);
#2240=LINE('',#12236,#3112);
#2241=LINE('',#12237,#3113);
#2242=LINE('',#12239,#3114);
#2713=VECTOR('',#9239,1.);
#2714=VECTOR('',#9240,1.);
#2715=VECTOR('',#9241,1.);
#2716=VECTOR('',#9242,1.);
#2717=VECTOR('',#9243,1.);
#2718=VECTOR('',#9244,1.);
#2719=VECTOR('',#9245,1.);
#2720=VECTOR('',#9246,1.);
#2721=VECTOR('',#9249,1.);
#2722=VECTOR('',#9250,1.);
#2723=VECTOR('',#9251,1.);
#2724=VECTOR('',#9252,1.);
#2725=VECTOR('',#9253,1.);
#2726=VECTOR('',#9254,1.);
#2727=VECTOR('',#9255,1.);
#2728=VECTOR('',#9256,1.);
#2729=VECTOR('',#9259,1.);
#2730=VECTOR('',#9260,1.);
#2731=VECTOR('',#9261,1.);
#2732=VECTOR('',#9262,1.);
#2733=VECTOR('',#9263,1.);
#2734=VECTOR('',#9264,1.);
#2735=VECTOR('',#9265,1.);
#2736=VECTOR('',#9266,1.);
#2737=VECTOR('',#9269,1.);
#2738=VECTOR('',#9270,1.);
#2739=VECTOR('',#9271,1.);
#2740=VECTOR('',#9272,1.);
#2741=VECTOR('',#9273,1.);
#2742=VECTOR('',#9274,1.);
#2743=VECTOR('',#9275,1.);
#2744=VECTOR('',#9276,1.);
#2745=VECTOR('',#9279,1.);
#2746=VECTOR('',#9280,1.);
#2747=VECTOR('',#9281,1.);
#2748=VECTOR('',#9282,1.);
#2749=VECTOR('',#9283,1.);
#2750=VECTOR('',#9284,1.);
#2751=VECTOR('',#9285,1.);
#2752=VECTOR('',#9286,1.);
#2753=VECTOR('',#9289,1.);
#2754=VECTOR('',#9290,1.);
#2755=VECTOR('',#9291,1.);
#2756=VECTOR('',#9292,1.);
#2757=VECTOR('',#9293,1.);
#2758=VECTOR('',#9294,1.);
#2759=VECTOR('',#9295,1.);
#2760=VECTOR('',#9296,1.);
#2761=VECTOR('',#9301,1.);
#2762=VECTOR('',#9304,1.);
#2763=VECTOR('',#9307,1.);
#2764=VECTOR('',#9310,1.);
#2765=VECTOR('',#9313,1.);
#2766=VECTOR('',#9316,1.);
#2767=VECTOR('',#9319,1.);
#2768=VECTOR('',#9320,1.);
#2769=VECTOR('',#9325,1.);
#2770=VECTOR('',#9326,1.);
#2771=VECTOR('',#9331,1.);
#2772=VECTOR('',#9332,1.);
#2773=VECTOR('',#9337,1.);
#2774=VECTOR('',#9338,1.);
#2775=VECTOR('',#9339,1.);
#2776=VECTOR('',#9340,1.);
#2777=VECTOR('',#9341,1.);
#2778=VECTOR('',#9342,1.);
#2779=VECTOR('',#9343,1.);
#2780=VECTOR('',#9344,1.);
#2781=VECTOR('',#9345,1.);
#2782=VECTOR('',#9346,1.);
#2783=VECTOR('',#9347,1.);
#2784=VECTOR('',#9348,1.);
#2785=VECTOR('',#9349,1.);
#2786=VECTOR('',#9350,1.);
#2787=VECTOR('',#9351,1.);
#2788=VECTOR('',#9352,1.);
#2789=VECTOR('',#9353,1.);
#2790=VECTOR('',#9354,1.);
#2791=VECTOR('',#9355,1.);
#2792=VECTOR('',#9356,1.);
#2793=VECTOR('',#9357,1.);
#2794=VECTOR('',#9358,1.);
#2795=VECTOR('',#9359,1.);
#2796=VECTOR('',#9360,1.);
#2797=VECTOR('',#9361,1.);
#2798=VECTOR('',#9362,1.);
#2799=VECTOR('',#9363,1.);
#2800=VECTOR('',#9364,1.);
#2801=VECTOR('',#9365,1.);
#2802=VECTOR('',#9366,1.);
#2803=VECTOR('',#9367,1.);
#2804=VECTOR('',#9368,1.);
#2805=VECTOR('',#9369,1.);
#2806=VECTOR('',#9370,1.);
#2807=VECTOR('',#9371,1.);
#2808=VECTOR('',#9372,1.);
#2809=VECTOR('',#9373,1.);
#2810=VECTOR('',#9374,1.);
#2811=VECTOR('',#9375,1.);
#2812=VECTOR('',#9376,1.);
#2813=VECTOR('',#9377,1.);
#2814=VECTOR('',#9378,1.);
#2815=VECTOR('',#9379,1.);
#2816=VECTOR('',#9380,1.);
#2817=VECTOR('',#9381,1.);
#2818=VECTOR('',#9382,1.);
#2819=VECTOR('',#9383,1.);
#2820=VECTOR('',#9384,1.);
#2821=VECTOR('',#9387,1.);
#2822=VECTOR('',#9388,1.);
#2823=VECTOR('',#9389,1.);
#2824=VECTOR('',#9390,1.);
#2825=VECTOR('',#9391,1.);
#2826=VECTOR('',#9394,1.);
#2827=VECTOR('',#9395,1.);
#2828=VECTOR('',#9398,1.);
#2829=VECTOR('',#9399,1.);
#2830=VECTOR('',#9402,1.);
#2831=VECTOR('',#9403,1.);
#2832=VECTOR('',#9406,1.);
#2833=VECTOR('',#9407,1.);
#2834=VECTOR('',#9410,1.);
#2835=VECTOR('',#9411,1.);
#2836=VECTOR('',#9414,1.);
#2837=VECTOR('',#9415,1.);
#2838=VECTOR('',#9418,1.);
#2839=VECTOR('',#9419,1.);
#2840=VECTOR('',#9422,1.);
#2841=VECTOR('',#9423,1.);
#2842=VECTOR('',#9424,1.);
#2843=VECTOR('',#9425,1.);
#2844=VECTOR('',#9426,1.);
#2845=VECTOR('',#9427,1.);
#2846=VECTOR('',#9428,1.);
#2847=VECTOR('',#9429,1.);
#2848=VECTOR('',#9430,1.);
#2849=VECTOR('',#9431,1.);
#2850=VECTOR('',#9432,1.);
#2851=VECTOR('',#9433,1.);
#2852=VECTOR('',#9436,1.);
#2853=VECTOR('',#9437,1.);
#2854=VECTOR('',#9440,1.);
#2855=VECTOR('',#9443,1.);
#2856=VECTOR('',#9446,1.);
#2857=VECTOR('',#9451,1.);
#2858=VECTOR('',#9452,1.);
#2859=VECTOR('',#9455,1.);
#2860=VECTOR('',#9456,1.);
#2861=VECTOR('',#9459,1.);
#2862=VECTOR('',#9460,1.);
#2863=VECTOR('',#9463,1.);
#2864=VECTOR('',#9464,1.);
#2865=VECTOR('',#9467,1.);
#2866=VECTOR('',#9468,1.);
#2867=VECTOR('',#9471,1.);
#2868=VECTOR('',#9472,1.);
#2869=VECTOR('',#9475,1.);
#2870=VECTOR('',#9480,1.);
#2871=VECTOR('',#9481,1.);
#2872=VECTOR('',#9482,1.);
#2873=VECTOR('',#9483,1.);
#2874=VECTOR('',#9484,1.);
#2875=VECTOR('',#9487,1.);
#2876=VECTOR('',#9488,1.);
#2877=VECTOR('',#9491,1.);
#2878=VECTOR('',#9492,1.);
#2879=VECTOR('',#9495,1.);
#2880=VECTOR('',#9496,1.);
#2881=VECTOR('',#9499,1.);
#2882=VECTOR('',#9500,1.);
#2883=VECTOR('',#9503,1.);
#2884=VECTOR('',#9504,1.);
#2885=VECTOR('',#9507,1.);
#2886=VECTOR('',#9508,1.);
#2887=VECTOR('',#9511,1.);
#2888=VECTOR('',#9512,1.);
#2889=VECTOR('',#9515,1.);
#2890=VECTOR('',#9516,1.);
#2891=VECTOR('',#9517,1.);
#2892=VECTOR('',#9518,1.);
#2893=VECTOR('',#9519,1.);
#2894=VECTOR('',#9520,1.);
#2895=VECTOR('',#9521,1.);
#2896=VECTOR('',#9522,1.);
#2897=VECTOR('',#9523,1.);
#2898=VECTOR('',#9524,1.);
#2899=VECTOR('',#9525,1.);
#2900=VECTOR('',#9526,1.);
#2901=VECTOR('',#9529,1.);
#2902=VECTOR('',#9530,1.);
#2903=VECTOR('',#9533,1.);
#2904=VECTOR('',#9536,1.);
#2905=VECTOR('',#9539,1.);
#2906=VECTOR('',#9544,1.);
#2907=VECTOR('',#9545,1.);
#2908=VECTOR('',#9548,1.);
#2909=VECTOR('',#9549,1.);
#2910=VECTOR('',#9552,1.);
#2911=VECTOR('',#9553,1.);
#2912=VECTOR('',#9556,1.);
#2913=VECTOR('',#9557,1.);
#2914=VECTOR('',#9560,1.);
#2915=VECTOR('',#9561,1.);
#2916=VECTOR('',#9564,1.);
#2917=VECTOR('',#9565,1.);
#2918=VECTOR('',#9568,1.);
#2919=VECTOR('',#9573,1.);
#2920=VECTOR('',#9574,1.);
#2921=VECTOR('',#9575,1.);
#2922=VECTOR('',#9576,1.);
#2923=VECTOR('',#9577,1.);
#2924=VECTOR('',#9580,1.);
#2925=VECTOR('',#9581,1.);
#2926=VECTOR('',#9584,1.);
#2927=VECTOR('',#9585,1.);
#2928=VECTOR('',#9588,1.);
#2929=VECTOR('',#9589,1.);
#2930=VECTOR('',#9592,1.);
#2931=VECTOR('',#9593,1.);
#2932=VECTOR('',#9596,1.);
#2933=VECTOR('',#9597,1.);
#2934=VECTOR('',#9600,1.);
#2935=VECTOR('',#9601,1.);
#2936=VECTOR('',#9604,1.);
#2937=VECTOR('',#9605,1.);
#2938=VECTOR('',#9608,1.);
#2939=VECTOR('',#9609,1.);
#2940=VECTOR('',#9610,1.);
#2941=VECTOR('',#9611,1.);
#2942=VECTOR('',#9612,1.);
#2943=VECTOR('',#9613,1.);
#2944=VECTOR('',#9614,1.);
#2945=VECTOR('',#9615,1.);
#2946=VECTOR('',#9616,1.);
#2947=VECTOR('',#9617,1.);
#2948=VECTOR('',#9618,1.);
#2949=VECTOR('',#9619,1.);
#2950=VECTOR('',#9622,1.);
#2951=VECTOR('',#9623,1.);
#2952=VECTOR('',#9626,1.);
#2953=VECTOR('',#9629,1.);
#2954=VECTOR('',#9632,1.);
#2955=VECTOR('',#9637,1.);
#2956=VECTOR('',#9638,1.);
#2957=VECTOR('',#9641,1.);
#2958=VECTOR('',#9642,1.);
#2959=VECTOR('',#9645,1.);
#2960=VECTOR('',#9646,1.);
#2961=VECTOR('',#9649,1.);
#2962=VECTOR('',#9650,1.);
#2963=VECTOR('',#9653,1.);
#2964=VECTOR('',#9654,1.);
#2965=VECTOR('',#9657,1.);
#2966=VECTOR('',#9658,1.);
#2967=VECTOR('',#9661,1.);
#2968=VECTOR('',#9666,1.);
#2969=VECTOR('',#9667,1.);
#2970=VECTOR('',#9668,1.);
#2971=VECTOR('',#9669,1.);
#2972=VECTOR('',#9670,1.);
#2973=VECTOR('',#9673,1.);
#2974=VECTOR('',#9674,1.);
#2975=VECTOR('',#9677,1.);
#2976=VECTOR('',#9678,1.);
#2977=VECTOR('',#9681,1.);
#2978=VECTOR('',#9682,1.);
#2979=VECTOR('',#9685,1.);
#2980=VECTOR('',#9686,1.);
#2981=VECTOR('',#9689,1.);
#2982=VECTOR('',#9690,1.);
#2983=VECTOR('',#9693,1.);
#2984=VECTOR('',#9694,1.);
#2985=VECTOR('',#9697,1.);
#2986=VECTOR('',#9698,1.);
#2987=VECTOR('',#9701,1.);
#2988=VECTOR('',#9702,1.);
#2989=VECTOR('',#9703,1.);
#2990=VECTOR('',#9704,1.);
#2991=VECTOR('',#9705,1.);
#2992=VECTOR('',#9706,1.);
#2993=VECTOR('',#9707,1.);
#2994=VECTOR('',#9708,1.);
#2995=VECTOR('',#9709,1.);
#2996=VECTOR('',#9710,1.);
#2997=VECTOR('',#9711,1.);
#2998=VECTOR('',#9712,1.);
#2999=VECTOR('',#9715,1.);
#3000=VECTOR('',#9716,1.);
#3001=VECTOR('',#9719,1.);
#3002=VECTOR('',#9722,1.);
#3003=VECTOR('',#9725,1.);
#3004=VECTOR('',#9730,1.);
#3005=VECTOR('',#9731,1.);
#3006=VECTOR('',#9734,1.);
#3007=VECTOR('',#9735,1.);
#3008=VECTOR('',#9738,1.);
#3009=VECTOR('',#9739,1.);
#3010=VECTOR('',#9742,1.);
#3011=VECTOR('',#9743,1.);
#3012=VECTOR('',#9746,1.);
#3013=VECTOR('',#9747,1.);
#3014=VECTOR('',#9750,1.);
#3015=VECTOR('',#9751,1.);
#3016=VECTOR('',#9754,1.);
#3017=VECTOR('',#9759,1.);
#3018=VECTOR('',#9760,1.);
#3019=VECTOR('',#9761,1.);
#3020=VECTOR('',#9762,1.);
#3021=VECTOR('',#9763,1.);
#3022=VECTOR('',#9766,1.);
#3023=VECTOR('',#9767,1.);
#3024=VECTOR('',#9770,1.);
#3025=VECTOR('',#9771,1.);
#3026=VECTOR('',#9774,1.);
#3027=VECTOR('',#9775,1.);
#3028=VECTOR('',#9778,1.);
#3029=VECTOR('',#9779,1.);
#3030=VECTOR('',#9782,1.);
#3031=VECTOR('',#9783,1.);
#3032=VECTOR('',#9786,1.);
#3033=VECTOR('',#9787,1.);
#3034=VECTOR('',#9790,1.);
#3035=VECTOR('',#9791,1.);
#3036=VECTOR('',#9794,1.);
#3037=VECTOR('',#9795,1.);
#3038=VECTOR('',#9796,1.);
#3039=VECTOR('',#9797,1.);
#3040=VECTOR('',#9798,1.);
#3041=VECTOR('',#9799,1.);
#3042=VECTOR('',#9800,1.);
#3043=VECTOR('',#9801,1.);
#3044=VECTOR('',#9802,1.);
#3045=VECTOR('',#9803,1.);
#3046=VECTOR('',#9804,1.);
#3047=VECTOR('',#9805,1.);
#3048=VECTOR('',#9808,1.);
#3049=VECTOR('',#9809,1.);
#3050=VECTOR('',#9812,1.);
#3051=VECTOR('',#9815,1.);
#3052=VECTOR('',#9818,1.);
#3053=VECTOR('',#9823,1.);
#3054=VECTOR('',#9824,1.);
#3055=VECTOR('',#9827,1.);
#3056=VECTOR('',#9828,1.);
#3057=VECTOR('',#9831,1.);
#3058=VECTOR('',#9832,1.);
#3059=VECTOR('',#9835,1.);
#3060=VECTOR('',#9836,1.);
#3061=VECTOR('',#9839,1.);
#3062=VECTOR('',#9840,1.);
#3063=VECTOR('',#9843,1.);
#3064=VECTOR('',#9844,1.);
#3065=VECTOR('',#9847,1.);
#3066=VECTOR('',#9852,1.);
#3067=VECTOR('',#9853,1.);
#3068=VECTOR('',#9854,1.);
#3069=VECTOR('',#9855,1.);
#3070=VECTOR('',#9856,1.);
#3071=VECTOR('',#9859,1.);
#3072=VECTOR('',#9860,1.);
#3073=VECTOR('',#9863,1.);
#3074=VECTOR('',#9864,1.);
#3075=VECTOR('',#9867,1.);
#3076=VECTOR('',#9868,1.);
#3077=VECTOR('',#9871,1.);
#3078=VECTOR('',#9872,1.);
#3079=VECTOR('',#9875,1.);
#3080=VECTOR('',#9876,1.);
#3081=VECTOR('',#9879,1.);
#3082=VECTOR('',#9880,1.);
#3083=VECTOR('',#9883,1.);
#3084=VECTOR('',#9884,1.);
#3085=VECTOR('',#9887,1.);
#3086=VECTOR('',#9888,1.);
#3087=VECTOR('',#9889,1.);
#3088=VECTOR('',#9890,1.);
#3089=VECTOR('',#9891,1.);
#3090=VECTOR('',#9892,1.);
#3091=VECTOR('',#9893,1.);
#3092=VECTOR('',#9894,1.);
#3093=VECTOR('',#9895,1.);
#3094=VECTOR('',#9896,1.);
#3095=VECTOR('',#9897,1.);
#3096=VECTOR('',#9898,1.);
#3097=VECTOR('',#9901,1.);
#3098=VECTOR('',#9902,1.);
#3099=VECTOR('',#9905,1.);
#3100=VECTOR('',#9908,1.);
#3101=VECTOR('',#9911,1.);
#3102=VECTOR('',#9916,1.);
#3103=VECTOR('',#9917,1.);
#3104=VECTOR('',#9920,1.);
#3105=VECTOR('',#9921,1.);
#3106=VECTOR('',#9924,1.);
#3107=VECTOR('',#9925,1.);
#3108=VECTOR('',#9928,1.);
#3109=VECTOR('',#9929,1.);
#3110=VECTOR('',#9932,1.);
#3111=VECTOR('',#9933,1.);
#3112=VECTOR('',#9936,1.);
#3113=VECTOR('',#9937,1.);
#3114=VECTOR('',#9940,1.);
#3245=CIRCLE('',#7855,0.817);
#3246=CIRCLE('',#7856,0.817);
#3247=CIRCLE('',#7857,0.817);
#3248=CIRCLE('',#7858,0.817);
#3249=CIRCLE('',#7859,0.817);
#3250=CIRCLE('',#7860,0.817);
#3251=CIRCLE('',#7862,0.817);
#3252=CIRCLE('',#7864,0.817);
#3253=CIRCLE('',#7866,0.817);
#3254=CIRCLE('',#7868,0.817);
#3255=CIRCLE('',#7870,0.817);
#3256=CIRCLE('',#7872,0.817);
#3601=VERTEX_POINT('',#11412);
#3602=VERTEX_POINT('',#11413);
#3603=VERTEX_POINT('',#11415);
#3604=VERTEX_POINT('',#11417);
#3605=VERTEX_POINT('',#11419);
#3606=VERTEX_POINT('',#11421);
#3607=VERTEX_POINT('',#11423);
#3608=VERTEX_POINT('',#11425);
#3609=VERTEX_POINT('',#11427);
#3610=VERTEX_POINT('',#11429);
#3611=VERTEX_POINT('',#11431);
#3612=VERTEX_POINT('',#11433);
#3613=VERTEX_POINT('',#11435);
#3614=VERTEX_POINT('',#11437);
#3615=VERTEX_POINT('',#11439);
#3616=VERTEX_POINT('',#11441);
#3617=VERTEX_POINT('',#11443);
#3618=VERTEX_POINT('',#11445);
#3619=VERTEX_POINT('',#11447);
#3620=VERTEX_POINT('',#11449);
#3621=VERTEX_POINT('',#11451);
#3622=VERTEX_POINT('',#11453);
#3623=VERTEX_POINT('',#11455);
#3624=VERTEX_POINT('',#11457);
#3625=VERTEX_POINT('',#11459);
#3626=VERTEX_POINT('',#11461);
#3627=VERTEX_POINT('',#11463);
#3628=VERTEX_POINT('',#11465);
#3629=VERTEX_POINT('',#11467);
#3630=VERTEX_POINT('',#11469);
#3631=VERTEX_POINT('',#11471);
#3632=VERTEX_POINT('',#11473);
#3633=VERTEX_POINT('',#11475);
#3634=VERTEX_POINT('',#11477);
#3635=VERTEX_POINT('',#11479);
#3636=VERTEX_POINT('',#11481);
#3637=VERTEX_POINT('',#11483);
#3638=VERTEX_POINT('',#11485);
#3639=VERTEX_POINT('',#11487);
#3640=VERTEX_POINT('',#11489);
#3641=VERTEX_POINT('',#11491);
#3642=VERTEX_POINT('',#11493);
#3643=VERTEX_POINT('',#11495);
#3644=VERTEX_POINT('',#11497);
#3645=VERTEX_POINT('',#11499);
#3646=VERTEX_POINT('',#11501);
#3647=VERTEX_POINT('',#11503);
#3648=VERTEX_POINT('',#11505);
#3649=VERTEX_POINT('',#11507);
#3650=VERTEX_POINT('',#11509);
#3651=VERTEX_POINT('',#11511);
#3652=VERTEX_POINT('',#11513);
#3653=VERTEX_POINT('',#11515);
#3654=VERTEX_POINT('',#11517);
#3655=VERTEX_POINT('',#11521);
#3656=VERTEX_POINT('',#11523);
#3657=VERTEX_POINT('',#11527);
#3658=VERTEX_POINT('',#11529);
#3659=VERTEX_POINT('',#11533);
#3660=VERTEX_POINT('',#11535);
#3661=VERTEX_POINT('',#11539);
#3662=VERTEX_POINT('',#11541);
#3663=VERTEX_POINT('',#11545);
#3664=VERTEX_POINT('',#11547);
#3665=VERTEX_POINT('',#11551);
#3666=VERTEX_POINT('',#11553);
#3667=VERTEX_POINT('',#11557);
#3668=VERTEX_POINT('',#11559);
#3669=VERTEX_POINT('',#11561);
#3670=VERTEX_POINT('',#11563);
#3671=VERTEX_POINT('',#11565);
#3672=VERTEX_POINT('',#11567);
#3673=VERTEX_POINT('',#11569);
#3674=VERTEX_POINT('',#11571);
#3675=VERTEX_POINT('',#11574);
#3676=VERTEX_POINT('',#11576);
#3677=VERTEX_POINT('',#11578);
#3678=VERTEX_POINT('',#11580);
#3679=VERTEX_POINT('',#11582);
#3680=VERTEX_POINT('',#11584);
#3681=VERTEX_POINT('',#11586);
#3682=VERTEX_POINT('',#11589);
#3683=VERTEX_POINT('',#11591);
#3684=VERTEX_POINT('',#11593);
#3685=VERTEX_POINT('',#11595);
#3686=VERTEX_POINT('',#11597);
#3687=VERTEX_POINT('',#11599);
#3688=VERTEX_POINT('',#11601);
#3689=VERTEX_POINT('',#11604);
#3690=VERTEX_POINT('',#11606);
#3691=VERTEX_POINT('',#11608);
#3692=VERTEX_POINT('',#11610);
#3693=VERTEX_POINT('',#11612);
#3694=VERTEX_POINT('',#11614);
#3695=VERTEX_POINT('',#11616);
#3696=VERTEX_POINT('',#11619);
#3697=VERTEX_POINT('',#11621);
#3698=VERTEX_POINT('',#11623);
#3699=VERTEX_POINT('',#11625);
#3700=VERTEX_POINT('',#11627);
#3701=VERTEX_POINT('',#11629);
#3702=VERTEX_POINT('',#11631);
#3703=VERTEX_POINT('',#11634);
#3704=VERTEX_POINT('',#11636);
#3705=VERTEX_POINT('',#11638);
#3706=VERTEX_POINT('',#11640);
#3707=VERTEX_POINT('',#11642);
#3708=VERTEX_POINT('',#11644);
#3709=VERTEX_POINT('',#11648);
#3710=VERTEX_POINT('',#11650);
#3711=VERTEX_POINT('',#11652);
#3712=VERTEX_POINT('',#11654);
#3713=VERTEX_POINT('',#11658);
#3714=VERTEX_POINT('',#11662);
#3715=VERTEX_POINT('',#11666);
#3716=VERTEX_POINT('',#11670);
#3717=VERTEX_POINT('',#11674);
#3718=VERTEX_POINT('',#11678);
#3719=VERTEX_POINT('',#11682);
#3720=VERTEX_POINT('',#11686);
#3721=VERTEX_POINT('',#11687);
#3722=VERTEX_POINT('',#11689);
#3723=VERTEX_POINT('',#11691);
#3724=VERTEX_POINT('',#11693);
#3725=VERTEX_POINT('',#11695);
#3726=VERTEX_POINT('',#11698);
#3727=VERTEX_POINT('',#11700);
#3728=VERTEX_POINT('',#11702);
#3729=VERTEX_POINT('',#11704);
#3730=VERTEX_POINT('',#11706);
#3731=VERTEX_POINT('',#11720);
#3732=VERTEX_POINT('',#11724);
#3733=VERTEX_POINT('',#11728);
#3734=VERTEX_POINT('',#11732);
#3735=VERTEX_POINT('',#11736);
#3736=VERTEX_POINT('',#11740);
#3737=VERTEX_POINT('',#11747);
#3738=VERTEX_POINT('',#11749);
#3739=VERTEX_POINT('',#11751);
#3740=VERTEX_POINT('',#11753);
#3741=VERTEX_POINT('',#11757);
#3742=VERTEX_POINT('',#11761);
#3743=VERTEX_POINT('',#11765);
#3744=VERTEX_POINT('',#11769);
#3745=VERTEX_POINT('',#11773);
#3746=VERTEX_POINT('',#11777);
#3747=VERTEX_POINT('',#11781);
#3748=VERTEX_POINT('',#11785);
#3749=VERTEX_POINT('',#11786);
#3750=VERTEX_POINT('',#11788);
#3751=VERTEX_POINT('',#11790);
#3752=VERTEX_POINT('',#11792);
#3753=VERTEX_POINT('',#11794);
#3754=VERTEX_POINT('',#11797);
#3755=VERTEX_POINT('',#11799);
#3756=VERTEX_POINT('',#11801);
#3757=VERTEX_POINT('',#11803);
#3758=VERTEX_POINT('',#11805);
#3759=VERTEX_POINT('',#11819);
#3760=VERTEX_POINT('',#11823);
#3761=VERTEX_POINT('',#11827);
#3762=VERTEX_POINT('',#11831);
#3763=VERTEX_POINT('',#11835);
#3764=VERTEX_POINT('',#11839);
#3765=VERTEX_POINT('',#11846);
#3766=VERTEX_POINT('',#11848);
#3767=VERTEX_POINT('',#11850);
#3768=VERTEX_POINT('',#11852);
#3769=VERTEX_POINT('',#11856);
#3770=VERTEX_POINT('',#11860);
#3771=VERTEX_POINT('',#11864);
#3772=VERTEX_POINT('',#11868);
#3773=VERTEX_POINT('',#11872);
#3774=VERTEX_POINT('',#11876);
#3775=VERTEX_POINT('',#11880);
#3776=VERTEX_POINT('',#11884);
#3777=VERTEX_POINT('',#11885);
#3778=VERTEX_POINT('',#11887);
#3779=VERTEX_POINT('',#11889);
#3780=VERTEX_POINT('',#11891);
#3781=VERTEX_POINT('',#11893);
#3782=VERTEX_POINT('',#11896);
#3783=VERTEX_POINT('',#11898);
#3784=VERTEX_POINT('',#11900);
#3785=VERTEX_POINT('',#11902);
#3786=VERTEX_POINT('',#11904);
#3787=VERTEX_POINT('',#11918);
#3788=VERTEX_POINT('',#11922);
#3789=VERTEX_POINT('',#11926);
#3790=VERTEX_POINT('',#11930);
#3791=VERTEX_POINT('',#11934);
#3792=VERTEX_POINT('',#11938);
#3793=VERTEX_POINT('',#11945);
#3794=VERTEX_POINT('',#11947);
#3795=VERTEX_POINT('',#11949);
#3796=VERTEX_POINT('',#11951);
#3797=VERTEX_POINT('',#11955);
#3798=VERTEX_POINT('',#11959);
#3799=VERTEX_POINT('',#11963);
#3800=VERTEX_POINT('',#11967);
#3801=VERTEX_POINT('',#11971);
#3802=VERTEX_POINT('',#11975);
#3803=VERTEX_POINT('',#11979);
#3804=VERTEX_POINT('',#11983);
#3805=VERTEX_POINT('',#11984);
#3806=VERTEX_POINT('',#11986);
#3807=VERTEX_POINT('',#11988);
#3808=VERTEX_POINT('',#11990);
#3809=VERTEX_POINT('',#11992);
#3810=VERTEX_POINT('',#11995);
#3811=VERTEX_POINT('',#11997);
#3812=VERTEX_POINT('',#11999);
#3813=VERTEX_POINT('',#12001);
#3814=VERTEX_POINT('',#12003);
#3815=VERTEX_POINT('',#12017);
#3816=VERTEX_POINT('',#12021);
#3817=VERTEX_POINT('',#12025);
#3818=VERTEX_POINT('',#12029);
#3819=VERTEX_POINT('',#12033);
#3820=VERTEX_POINT('',#12037);
#3821=VERTEX_POINT('',#12044);
#3822=VERTEX_POINT('',#12046);
#3823=VERTEX_POINT('',#12048);
#3824=VERTEX_POINT('',#12050);
#3825=VERTEX_POINT('',#12054);
#3826=VERTEX_POINT('',#12058);
#3827=VERTEX_POINT('',#12062);
#3828=VERTEX_POINT('',#12066);
#3829=VERTEX_POINT('',#12070);
#3830=VERTEX_POINT('',#12074);
#3831=VERTEX_POINT('',#12078);
#3832=VERTEX_POINT('',#12082);
#3833=VERTEX_POINT('',#12083);
#3834=VERTEX_POINT('',#12085);
#3835=VERTEX_POINT('',#12087);
#3836=VERTEX_POINT('',#12089);
#3837=VERTEX_POINT('',#12091);
#3838=VERTEX_POINT('',#12094);
#3839=VERTEX_POINT('',#12096);
#3840=VERTEX_POINT('',#12098);
#3841=VERTEX_POINT('',#12100);
#3842=VERTEX_POINT('',#12102);
#3843=VERTEX_POINT('',#12116);
#3844=VERTEX_POINT('',#12120);
#3845=VERTEX_POINT('',#12124);
#3846=VERTEX_POINT('',#12128);
#3847=VERTEX_POINT('',#12132);
#3848=VERTEX_POINT('',#12136);
#3849=VERTEX_POINT('',#12143);
#3850=VERTEX_POINT('',#12145);
#3851=VERTEX_POINT('',#12147);
#3852=VERTEX_POINT('',#12149);
#3853=VERTEX_POINT('',#12153);
#3854=VERTEX_POINT('',#12157);
#3855=VERTEX_POINT('',#12161);
#3856=VERTEX_POINT('',#12165);
#3857=VERTEX_POINT('',#12169);
#3858=VERTEX_POINT('',#12173);
#3859=VERTEX_POINT('',#12177);
#3860=VERTEX_POINT('',#12181);
#3861=VERTEX_POINT('',#12182);
#3862=VERTEX_POINT('',#12184);
#3863=VERTEX_POINT('',#12186);
#3864=VERTEX_POINT('',#12188);
#3865=VERTEX_POINT('',#12190);
#3866=VERTEX_POINT('',#12193);
#3867=VERTEX_POINT('',#12195);
#3868=VERTEX_POINT('',#12197);
#3869=VERTEX_POINT('',#12199);
#3870=VERTEX_POINT('',#12201);
#3871=VERTEX_POINT('',#12215);
#3872=VERTEX_POINT('',#12219);
#3873=VERTEX_POINT('',#12223);
#3874=VERTEX_POINT('',#12227);
#3875=VERTEX_POINT('',#12231);
#3876=VERTEX_POINT('',#12235);
#4460=EDGE_CURVE('',#3601,#3602,#1841,.T.);
#4461=EDGE_CURVE('',#3603,#3601,#1842,.T.);
#4462=EDGE_CURVE('',#3604,#3603,#1843,.T.);
#4463=EDGE_CURVE('',#3605,#3604,#1844,.T.);
#4464=EDGE_CURVE('',#3606,#3605,#1845,.T.);
#4465=EDGE_CURVE('',#3607,#3606,#1846,.T.);
#4466=EDGE_CURVE('',#3608,#3607,#1847,.T.);
#4467=EDGE_CURVE('',#3609,#3608,#1848,.T.);
#4468=EDGE_CURVE('',#3609,#3610,#3245,.T.);
#4469=EDGE_CURVE('',#3611,#3610,#1849,.T.);
#4470=EDGE_CURVE('',#3612,#3611,#1850,.T.);
#4471=EDGE_CURVE('',#3613,#3612,#1851,.T.);
#4472=EDGE_CURVE('',#3614,#3613,#1852,.T.);
#4473=EDGE_CURVE('',#3615,#3614,#1853,.T.);
#4474=EDGE_CURVE('',#3616,#3615,#1854,.T.);
#4475=EDGE_CURVE('',#3617,#3616,#1855,.T.);
#4476=EDGE_CURVE('',#3618,#3617,#1856,.T.);
#4477=EDGE_CURVE('',#3618,#3619,#3246,.T.);
#4478=EDGE_CURVE('',#3620,#3619,#1857,.T.);
#4479=EDGE_CURVE('',#3621,#3620,#1858,.T.);
#4480=EDGE_CURVE('',#3622,#3621,#1859,.T.);
#4481=EDGE_CURVE('',#3623,#3622,#1860,.T.);
#4482=EDGE_CURVE('',#3624,#3623,#1861,.T.);
#4483=EDGE_CURVE('',#3625,#3624,#1862,.T.);
#4484=EDGE_CURVE('',#3626,#3625,#1863,.T.);
#4485=EDGE_CURVE('',#3627,#3626,#1864,.T.);
#4486=EDGE_CURVE('',#3627,#3628,#3247,.T.);
#4487=EDGE_CURVE('',#3629,#3628,#1865,.T.);
#4488=EDGE_CURVE('',#3630,#3629,#1866,.T.);
#4489=EDGE_CURVE('',#3631,#3630,#1867,.T.);
#4490=EDGE_CURVE('',#3632,#3631,#1868,.T.);
#4491=EDGE_CURVE('',#3633,#3632,#1869,.T.);
#4492=EDGE_CURVE('',#3634,#3633,#1870,.T.);
#4493=EDGE_CURVE('',#3635,#3634,#1871,.T.);
#4494=EDGE_CURVE('',#3636,#3635,#1872,.T.);
#4495=EDGE_CURVE('',#3636,#3637,#3248,.T.);
#4496=EDGE_CURVE('',#3638,#3637,#1873,.T.);
#4497=EDGE_CURVE('',#3639,#3638,#1874,.T.);
#4498=EDGE_CURVE('',#3640,#3639,#1875,.T.);
#4499=EDGE_CURVE('',#3641,#3640,#1876,.T.);
#4500=EDGE_CURVE('',#3642,#3641,#1877,.T.);
#4501=EDGE_CURVE('',#3643,#3642,#1878,.T.);
#4502=EDGE_CURVE('',#3644,#3643,#1879,.T.);
#4503=EDGE_CURVE('',#3645,#3644,#1880,.T.);
#4504=EDGE_CURVE('',#3645,#3646,#3249,.T.);
#4505=EDGE_CURVE('',#3647,#3646,#1881,.T.);
#4506=EDGE_CURVE('',#3648,#3647,#1882,.T.);
#4507=EDGE_CURVE('',#3649,#3648,#1883,.T.);
#4508=EDGE_CURVE('',#3650,#3649,#1884,.T.);
#4509=EDGE_CURVE('',#3651,#3650,#1885,.T.);
#4510=EDGE_CURVE('',#3652,#3651,#1886,.T.);
#4511=EDGE_CURVE('',#3653,#3652,#1887,.T.);
#4512=EDGE_CURVE('',#3654,#3653,#1888,.T.);
#4513=EDGE_CURVE('',#3654,#3602,#3250,.T.);
#4514=EDGE_CURVE('',#3655,#3645,#1889,.T.);
#4515=EDGE_CURVE('',#3656,#3655,#3251,.T.);
#4516=EDGE_CURVE('',#3646,#3656,#1890,.T.);
#4517=EDGE_CURVE('',#3657,#3609,#1891,.T.);
#4518=EDGE_CURVE('',#3658,#3657,#3252,.T.);
#4519=EDGE_CURVE('',#3610,#3658,#1892,.T.);
#4520=EDGE_CURVE('',#3659,#3627,#1893,.T.);
#4521=EDGE_CURVE('',#3660,#3659,#3253,.T.);
#4522=EDGE_CURVE('',#3628,#3660,#1894,.T.);
#4523=EDGE_CURVE('',#3637,#3661,#1895,.T.);
#4524=EDGE_CURVE('',#3662,#3636,#1896,.T.);
#4525=EDGE_CURVE('',#3661,#3662,#3254,.T.);
#4526=EDGE_CURVE('',#3619,#3663,#1897,.T.);
#4527=EDGE_CURVE('',#3664,#3618,#1898,.T.);
#4528=EDGE_CURVE('',#3663,#3664,#3255,.T.);
#4529=EDGE_CURVE('',#3602,#3665,#1899,.T.);
#4530=EDGE_CURVE('',#3666,#3654,#1900,.T.);
#4531=EDGE_CURVE('',#3665,#3666,#3256,.T.);
#4532=EDGE_CURVE('',#3665,#3667,#1901,.T.);
#4533=EDGE_CURVE('',#3668,#3666,#1902,.T.);
#4534=EDGE_CURVE('',#3669,#3668,#1903,.T.);
#4535=EDGE_CURVE('',#3670,#3669,#1904,.T.);
#4536=EDGE_CURVE('',#3671,#3670,#1905,.T.);
#4537=EDGE_CURVE('',#3672,#3671,#1906,.T.);
#4538=EDGE_CURVE('',#3673,#3672,#1907,.T.);
#4539=EDGE_CURVE('',#3674,#3673,#1908,.T.);
#4540=EDGE_CURVE('',#3656,#3674,#1909,.T.);
#4541=EDGE_CURVE('',#3675,#3655,#1910,.T.);
#4542=EDGE_CURVE('',#3676,#3675,#1911,.T.);
#4543=EDGE_CURVE('',#3677,#3676,#1912,.T.);
#4544=EDGE_CURVE('',#3678,#3677,#1913,.T.);
#4545=EDGE_CURVE('',#3679,#3678,#1914,.T.);
#4546=EDGE_CURVE('',#3680,#3679,#1915,.T.);
#4547=EDGE_CURVE('',#3681,#3680,#1916,.T.);
#4548=EDGE_CURVE('',#3661,#3681,#1917,.T.);
#4549=EDGE_CURVE('',#3682,#3662,#1918,.T.);
#4550=EDGE_CURVE('',#3683,#3682,#1919,.T.);
#4551=EDGE_CURVE('',#3684,#3683,#1920,.T.);
#4552=EDGE_CURVE('',#3685,#3684,#1921,.T.);
#4553=EDGE_CURVE('',#3686,#3685,#1922,.T.);
#4554=EDGE_CURVE('',#3687,#3686,#1923,.T.);
#4555=EDGE_CURVE('',#3688,#3687,#1924,.T.);
#4556=EDGE_CURVE('',#3660,#3688,#1925,.T.);
#4557=EDGE_CURVE('',#3689,#3659,#1926,.T.);
#4558=EDGE_CURVE('',#3690,#3689,#1927,.T.);
#4559=EDGE_CURVE('',#3691,#3690,#1928,.T.);
#4560=EDGE_CURVE('',#3692,#3691,#1929,.T.);
#4561=EDGE_CURVE('',#3693,#3692,#1930,.T.);
#4562=EDGE_CURVE('',#3694,#3693,#1931,.T.);
#4563=EDGE_CURVE('',#3695,#3694,#1932,.T.);
#4564=EDGE_CURVE('',#3663,#3695,#1933,.T.);
#4565=EDGE_CURVE('',#3696,#3664,#1934,.T.);
#4566=EDGE_CURVE('',#3697,#3696,#1935,.T.);
#4567=EDGE_CURVE('',#3698,#3697,#1936,.T.);
#4568=EDGE_CURVE('',#3699,#3698,#1937,.T.);
#4569=EDGE_CURVE('',#3700,#3699,#1938,.T.);
#4570=EDGE_CURVE('',#3701,#3700,#1939,.T.);
#4571=EDGE_CURVE('',#3702,#3701,#1940,.T.);
#4572=EDGE_CURVE('',#3658,#3702,#1941,.T.);
#4573=EDGE_CURVE('',#3703,#3657,#1942,.T.);
#4574=EDGE_CURVE('',#3704,#3703,#1943,.T.);
#4575=EDGE_CURVE('',#3705,#3704,#1944,.T.);
#4576=EDGE_CURVE('',#3706,#3705,#1945,.T.);
#4577=EDGE_CURVE('',#3707,#3706,#1946,.T.);
#4578=EDGE_CURVE('',#3708,#3707,#1947,.T.);
#4579=EDGE_CURVE('',#3667,#3708,#1948,.T.);
#4580=EDGE_CURVE('',#3674,#3709,#1949,.T.);
#4581=EDGE_CURVE('',#3710,#3709,#1950,.T.);
#4582=EDGE_CURVE('',#3711,#3710,#1951,.T.);
#4583=EDGE_CURVE('',#3712,#3711,#1952,.T.);
#4584=EDGE_CURVE('',#3712,#3647,#1953,.T.);
#4585=EDGE_CURVE('',#3673,#3713,#1954,.T.);
#4586=EDGE_CURVE('',#3709,#3713,#1955,.T.);
#4587=EDGE_CURVE('',#3714,#3712,#1956,.T.);
#4588=EDGE_CURVE('',#3714,#3648,#1957,.T.);
#4589=EDGE_CURVE('',#3672,#3715,#1958,.T.);
#4590=EDGE_CURVE('',#3713,#3715,#1959,.T.);
#4591=EDGE_CURVE('',#3671,#3716,#1960,.T.);
#4592=EDGE_CURVE('',#3715,#3716,#1961,.T.);
#4593=EDGE_CURVE('',#3670,#3717,#1962,.T.);
#4594=EDGE_CURVE('',#3716,#3717,#1963,.T.);
#4595=EDGE_CURVE('',#3669,#3718,#1964,.T.);
#4596=EDGE_CURVE('',#3717,#3718,#1965,.T.);
#4597=EDGE_CURVE('',#3719,#3668,#1966,.T.);
#4598=EDGE_CURVE('',#3718,#3719,#1967,.T.);
#4599=EDGE_CURVE('',#3720,#3721,#1968,.T.);
#4600=EDGE_CURVE('',#3721,#3722,#1969,.T.);
#4601=EDGE_CURVE('',#3722,#3723,#1970,.T.);
#4602=EDGE_CURVE('',#3723,#3724,#1971,.T.);
#4603=EDGE_CURVE('',#3724,#3725,#1972,.T.);
#4604=EDGE_CURVE('',#3725,#3714,#1973,.T.);
#4605=EDGE_CURVE('',#3711,#3726,#1974,.T.);
#4606=EDGE_CURVE('',#3726,#3727,#1975,.T.);
#4607=EDGE_CURVE('',#3727,#3728,#1976,.T.);
#4608=EDGE_CURVE('',#3728,#3729,#1977,.T.);
#4609=EDGE_CURVE('',#3729,#3730,#1978,.T.);
#4610=EDGE_CURVE('',#3730,#3720,#1979,.T.);
#4611=EDGE_CURVE('',#3722,#3652,#1980,.T.);
#4612=EDGE_CURVE('',#3653,#3721,#1981,.T.);
#4613=EDGE_CURVE('',#3723,#3651,#1982,.T.);
#4614=EDGE_CURVE('',#3724,#3650,#1983,.T.);
#4615=EDGE_CURVE('',#3725,#3649,#1984,.T.);
#4616=EDGE_CURVE('',#3731,#3710,#1985,.T.);
#4617=EDGE_CURVE('',#3726,#3731,#1986,.T.);
#4618=EDGE_CURVE('',#3732,#3731,#1987,.T.);
#4619=EDGE_CURVE('',#3727,#3732,#1988,.T.);
#4620=EDGE_CURVE('',#3733,#3732,#1989,.T.);
#4621=EDGE_CURVE('',#3728,#3733,#1990,.T.);
#4622=EDGE_CURVE('',#3734,#3733,#1991,.T.);
#4623=EDGE_CURVE('',#3729,#3734,#1992,.T.);
#4624=EDGE_CURVE('',#3735,#3734,#1993,.T.);
#4625=EDGE_CURVE('',#3730,#3735,#1994,.T.);
#4626=EDGE_CURVE('',#3736,#3735,#1995,.T.);
#4627=EDGE_CURVE('',#3720,#3736,#1996,.T.);
#4628=EDGE_CURVE('',#3719,#3736,#1997,.T.);
#4629=EDGE_CURVE('',#3702,#3737,#1998,.T.);
#4630=EDGE_CURVE('',#3738,#3737,#1999,.T.);
#4631=EDGE_CURVE('',#3739,#3738,#2000,.T.);
#4632=EDGE_CURVE('',#3740,#3739,#2001,.T.);
#4633=EDGE_CURVE('',#3740,#3611,#2002,.T.);
#4634=EDGE_CURVE('',#3701,#3741,#2003,.T.);
#4635=EDGE_CURVE('',#3737,#3741,#2004,.T.);
#4636=EDGE_CURVE('',#3742,#3740,#2005,.T.);
#4637=EDGE_CURVE('',#3742,#3612,#2006,.T.);
#4638=EDGE_CURVE('',#3700,#3743,#2007,.T.);
#4639=EDGE_CURVE('',#3741,#3743,#2008,.T.);
#4640=EDGE_CURVE('',#3699,#3744,#2009,.T.);
#4641=EDGE_CURVE('',#3743,#3744,#2010,.T.);
#4642=EDGE_CURVE('',#3698,#3745,#2011,.T.);
#4643=EDGE_CURVE('',#3744,#3745,#2012,.T.);
#4644=EDGE_CURVE('',#3697,#3746,#2013,.T.);
#4645=EDGE_CURVE('',#3745,#3746,#2014,.T.);
#4646=EDGE_CURVE('',#3747,#3696,#2015,.T.);
#4647=EDGE_CURVE('',#3746,#3747,#2016,.T.);
#4648=EDGE_CURVE('',#3748,#3749,#2017,.T.);
#4649=EDGE_CURVE('',#3749,#3750,#2018,.T.);
#4650=EDGE_CURVE('',#3750,#3751,#2019,.T.);
#4651=EDGE_CURVE('',#3751,#3752,#2020,.T.);
#4652=EDGE_CURVE('',#3752,#3753,#2021,.T.);
#4653=EDGE_CURVE('',#3753,#3742,#2022,.T.);
#4654=EDGE_CURVE('',#3739,#3754,#2023,.T.);
#4655=EDGE_CURVE('',#3754,#3755,#2024,.T.);
#4656=EDGE_CURVE('',#3755,#3756,#2025,.T.);
#4657=EDGE_CURVE('',#3756,#3757,#2026,.T.);
#4658=EDGE_CURVE('',#3757,#3758,#2027,.T.);
#4659=EDGE_CURVE('',#3758,#3748,#2028,.T.);
#4660=EDGE_CURVE('',#3750,#3616,#2029,.T.);
#4661=EDGE_CURVE('',#3617,#3749,#2030,.T.);
#4662=EDGE_CURVE('',#3751,#3615,#2031,.T.);
#4663=EDGE_CURVE('',#3752,#3614,#2032,.T.);
#4664=EDGE_CURVE('',#3753,#3613,#2033,.T.);
#4665=EDGE_CURVE('',#3759,#3738,#2034,.T.);
#4666=EDGE_CURVE('',#3754,#3759,#2035,.T.);
#4667=EDGE_CURVE('',#3760,#3759,#2036,.T.);
#4668=EDGE_CURVE('',#3755,#3760,#2037,.T.);
#4669=EDGE_CURVE('',#3761,#3760,#2038,.T.);
#4670=EDGE_CURVE('',#3756,#3761,#2039,.T.);
#4671=EDGE_CURVE('',#3762,#3761,#2040,.T.);
#4672=EDGE_CURVE('',#3757,#3762,#2041,.T.);
#4673=EDGE_CURVE('',#3763,#3762,#2042,.T.);
#4674=EDGE_CURVE('',#3758,#3763,#2043,.T.);
#4675=EDGE_CURVE('',#3764,#3763,#2044,.T.);
#4676=EDGE_CURVE('',#3748,#3764,#2045,.T.);
#4677=EDGE_CURVE('',#3747,#3764,#2046,.T.);
#4678=EDGE_CURVE('',#3688,#3765,#2047,.T.);
#4679=EDGE_CURVE('',#3766,#3765,#2048,.T.);
#4680=EDGE_CURVE('',#3767,#3766,#2049,.T.);
#4681=EDGE_CURVE('',#3768,#3767,#2050,.T.);
#4682=EDGE_CURVE('',#3768,#3629,#2051,.T.);
#4683=EDGE_CURVE('',#3687,#3769,#2052,.T.);
#4684=EDGE_CURVE('',#3765,#3769,#2053,.T.);
#4685=EDGE_CURVE('',#3770,#3768,#2054,.T.);
#4686=EDGE_CURVE('',#3770,#3630,#2055,.T.);
#4687=EDGE_CURVE('',#3686,#3771,#2056,.T.);
#4688=EDGE_CURVE('',#3769,#3771,#2057,.T.);
#4689=EDGE_CURVE('',#3685,#3772,#2058,.T.);
#4690=EDGE_CURVE('',#3771,#3772,#2059,.T.);
#4691=EDGE_CURVE('',#3684,#3773,#2060,.T.);
#4692=EDGE_CURVE('',#3772,#3773,#2061,.T.);
#4693=EDGE_CURVE('',#3683,#3774,#2062,.T.);
#4694=EDGE_CURVE('',#3773,#3774,#2063,.T.);
#4695=EDGE_CURVE('',#3775,#3682,#2064,.T.);
#4696=EDGE_CURVE('',#3774,#3775,#2065,.T.);
#4697=EDGE_CURVE('',#3776,#3777,#2066,.T.);
#4698=EDGE_CURVE('',#3777,#3778,#2067,.T.);
#4699=EDGE_CURVE('',#3778,#3779,#2068,.T.);
#4700=EDGE_CURVE('',#3779,#3780,#2069,.T.);
#4701=EDGE_CURVE('',#3780,#3781,#2070,.T.);
#4702=EDGE_CURVE('',#3781,#3770,#2071,.T.);
#4703=EDGE_CURVE('',#3767,#3782,#2072,.T.);
#4704=EDGE_CURVE('',#3782,#3783,#2073,.T.);
#4705=EDGE_CURVE('',#3783,#3784,#2074,.T.);
#4706=EDGE_CURVE('',#3784,#3785,#2075,.T.);
#4707=EDGE_CURVE('',#3785,#3786,#2076,.T.);
#4708=EDGE_CURVE('',#3786,#3776,#2077,.T.);
#4709=EDGE_CURVE('',#3778,#3634,#2078,.T.);
#4710=EDGE_CURVE('',#3635,#3777,#2079,.T.);
#4711=EDGE_CURVE('',#3779,#3633,#2080,.T.);
#4712=EDGE_CURVE('',#3780,#3632,#2081,.T.);
#4713=EDGE_CURVE('',#3781,#3631,#2082,.T.);
#4714=EDGE_CURVE('',#3787,#3766,#2083,.T.);
#4715=EDGE_CURVE('',#3782,#3787,#2084,.T.);
#4716=EDGE_CURVE('',#3788,#3787,#2085,.T.);
#4717=EDGE_CURVE('',#3783,#3788,#2086,.T.);
#4718=EDGE_CURVE('',#3789,#3788,#2087,.T.);
#4719=EDGE_CURVE('',#3784,#3789,#2088,.T.);
#4720=EDGE_CURVE('',#3790,#3789,#2089,.T.);
#4721=EDGE_CURVE('',#3785,#3790,#2090,.T.);
#4722=EDGE_CURVE('',#3791,#3790,#2091,.T.);
#4723=EDGE_CURVE('',#3786,#3791,#2092,.T.);
#4724=EDGE_CURVE('',#3792,#3791,#2093,.T.);
#4725=EDGE_CURVE('',#3776,#3792,#2094,.T.);
#4726=EDGE_CURVE('',#3775,#3792,#2095,.T.);
#4727=EDGE_CURVE('',#3681,#3793,#2096,.T.);
#4728=EDGE_CURVE('',#3794,#3793,#2097,.T.);
#4729=EDGE_CURVE('',#3795,#3794,#2098,.T.);
#4730=EDGE_CURVE('',#3796,#3795,#2099,.T.);
#4731=EDGE_CURVE('',#3796,#3638,#2100,.T.);
#4732=EDGE_CURVE('',#3680,#3797,#2101,.T.);
#4733=EDGE_CURVE('',#3793,#3797,#2102,.T.);
#4734=EDGE_CURVE('',#3798,#3796,#2103,.T.);
#4735=EDGE_CURVE('',#3798,#3639,#2104,.T.);
#4736=EDGE_CURVE('',#3679,#3799,#2105,.T.);
#4737=EDGE_CURVE('',#3797,#3799,#2106,.T.);
#4738=EDGE_CURVE('',#3678,#3800,#2107,.T.);
#4739=EDGE_CURVE('',#3799,#3800,#2108,.T.);
#4740=EDGE_CURVE('',#3677,#3801,#2109,.T.);
#4741=EDGE_CURVE('',#3800,#3801,#2110,.T.);
#4742=EDGE_CURVE('',#3676,#3802,#2111,.T.);
#4743=EDGE_CURVE('',#3801,#3802,#2112,.T.);
#4744=EDGE_CURVE('',#3803,#3675,#2113,.T.);
#4745=EDGE_CURVE('',#3802,#3803,#2114,.T.);
#4746=EDGE_CURVE('',#3804,#3805,#2115,.T.);
#4747=EDGE_CURVE('',#3805,#3806,#2116,.T.);
#4748=EDGE_CURVE('',#3806,#3807,#2117,.T.);
#4749=EDGE_CURVE('',#3807,#3808,#2118,.T.);
#4750=EDGE_CURVE('',#3808,#3809,#2119,.T.);
#4751=EDGE_CURVE('',#3809,#3798,#2120,.T.);
#4752=EDGE_CURVE('',#3795,#3810,#2121,.T.);
#4753=EDGE_CURVE('',#3810,#3811,#2122,.T.);
#4754=EDGE_CURVE('',#3811,#3812,#2123,.T.);
#4755=EDGE_CURVE('',#3812,#3813,#2124,.T.);
#4756=EDGE_CURVE('',#3813,#3814,#2125,.T.);
#4757=EDGE_CURVE('',#3814,#3804,#2126,.T.);
#4758=EDGE_CURVE('',#3806,#3643,#2127,.T.);
#4759=EDGE_CURVE('',#3644,#3805,#2128,.T.);
#4760=EDGE_CURVE('',#3807,#3642,#2129,.T.);
#4761=EDGE_CURVE('',#3808,#3641,#2130,.T.);
#4762=EDGE_CURVE('',#3809,#3640,#2131,.T.);
#4763=EDGE_CURVE('',#3815,#3794,#2132,.T.);
#4764=EDGE_CURVE('',#3810,#3815,#2133,.T.);
#4765=EDGE_CURVE('',#3816,#3815,#2134,.T.);
#4766=EDGE_CURVE('',#3811,#3816,#2135,.T.);
#4767=EDGE_CURVE('',#3817,#3816,#2136,.T.);
#4768=EDGE_CURVE('',#3812,#3817,#2137,.T.);
#4769=EDGE_CURVE('',#3818,#3817,#2138,.T.);
#4770=EDGE_CURVE('',#3813,#3818,#2139,.T.);
#4771=EDGE_CURVE('',#3819,#3818,#2140,.T.);
#4772=EDGE_CURVE('',#3814,#3819,#2141,.T.);
#4773=EDGE_CURVE('',#3820,#3819,#2142,.T.);
#4774=EDGE_CURVE('',#3804,#3820,#2143,.T.);
#4775=EDGE_CURVE('',#3803,#3820,#2144,.T.);
#4776=EDGE_CURVE('',#3695,#3821,#2145,.T.);
#4777=EDGE_CURVE('',#3822,#3821,#2146,.T.);
#4778=EDGE_CURVE('',#3823,#3822,#2147,.T.);
#4779=EDGE_CURVE('',#3824,#3823,#2148,.T.);
#4780=EDGE_CURVE('',#3824,#3620,#2149,.T.);
#4781=EDGE_CURVE('',#3694,#3825,#2150,.T.);
#4782=EDGE_CURVE('',#3821,#3825,#2151,.T.);
#4783=EDGE_CURVE('',#3826,#3824,#2152,.T.);
#4784=EDGE_CURVE('',#3826,#3621,#2153,.T.);
#4785=EDGE_CURVE('',#3693,#3827,#2154,.T.);
#4786=EDGE_CURVE('',#3825,#3827,#2155,.T.);
#4787=EDGE_CURVE('',#3692,#3828,#2156,.T.);
#4788=EDGE_CURVE('',#3827,#3828,#2157,.T.);
#4789=EDGE_CURVE('',#3691,#3829,#2158,.T.);
#4790=EDGE_CURVE('',#3828,#3829,#2159,.T.);
#4791=EDGE_CURVE('',#3690,#3830,#2160,.T.);
#4792=EDGE_CURVE('',#3829,#3830,#2161,.T.);
#4793=EDGE_CURVE('',#3831,#3689,#2162,.T.);
#4794=EDGE_CURVE('',#3830,#3831,#2163,.T.);
#4795=EDGE_CURVE('',#3832,#3833,#2164,.T.);
#4796=EDGE_CURVE('',#3833,#3834,#2165,.T.);
#4797=EDGE_CURVE('',#3834,#3835,#2166,.T.);
#4798=EDGE_CURVE('',#3835,#3836,#2167,.T.);
#4799=EDGE_CURVE('',#3836,#3837,#2168,.T.);
#4800=EDGE_CURVE('',#3837,#3826,#2169,.T.);
#4801=EDGE_CURVE('',#3823,#3838,#2170,.T.);
#4802=EDGE_CURVE('',#3838,#3839,#2171,.T.);
#4803=EDGE_CURVE('',#3839,#3840,#2172,.T.);
#4804=EDGE_CURVE('',#3840,#3841,#2173,.T.);
#4805=EDGE_CURVE('',#3841,#3842,#2174,.T.);
#4806=EDGE_CURVE('',#3842,#3832,#2175,.T.);
#4807=EDGE_CURVE('',#3834,#3625,#2176,.T.);
#4808=EDGE_CURVE('',#3626,#3833,#2177,.T.);
#4809=EDGE_CURVE('',#3835,#3624,#2178,.T.);
#4810=EDGE_CURVE('',#3836,#3623,#2179,.T.);
#4811=EDGE_CURVE('',#3837,#3622,#2180,.T.);
#4812=EDGE_CURVE('',#3843,#3822,#2181,.T.);
#4813=EDGE_CURVE('',#3838,#3843,#2182,.T.);
#4814=EDGE_CURVE('',#3844,#3843,#2183,.T.);
#4815=EDGE_CURVE('',#3839,#3844,#2184,.T.);
#4816=EDGE_CURVE('',#3845,#3844,#2185,.T.);
#4817=EDGE_CURVE('',#3840,#3845,#2186,.T.);
#4818=EDGE_CURVE('',#3846,#3845,#2187,.T.);
#4819=EDGE_CURVE('',#3841,#3846,#2188,.T.);
#4820=EDGE_CURVE('',#3847,#3846,#2189,.T.);
#4821=EDGE_CURVE('',#3842,#3847,#2190,.T.);
#4822=EDGE_CURVE('',#3848,#3847,#2191,.T.);
#4823=EDGE_CURVE('',#3832,#3848,#2192,.T.);
#4824=EDGE_CURVE('',#3831,#3848,#2193,.T.);
#4825=EDGE_CURVE('',#3667,#3849,#2194,.T.);
#4826=EDGE_CURVE('',#3850,#3849,#2195,.T.);
#4827=EDGE_CURVE('',#3851,#3850,#2196,.T.);
#4828=EDGE_CURVE('',#3852,#3851,#2197,.T.);
#4829=EDGE_CURVE('',#3852,#3601,#2198,.T.);
#4830=EDGE_CURVE('',#3708,#3853,#2199,.T.);
#4831=EDGE_CURVE('',#3849,#3853,#2200,.T.);
#4832=EDGE_CURVE('',#3854,#3852,#2201,.T.);
#4833=EDGE_CURVE('',#3854,#3603,#2202,.T.);
#4834=EDGE_CURVE('',#3707,#3855,#2203,.T.);
#4835=EDGE_CURVE('',#3853,#3855,#2204,.T.);
#4836=EDGE_CURVE('',#3706,#3856,#2205,.T.);
#4837=EDGE_CURVE('',#3855,#3856,#2206,.T.);
#4838=EDGE_CURVE('',#3705,#3857,#2207,.T.);
#4839=EDGE_CURVE('',#3856,#3857,#2208,.T.);
#4840=EDGE_CURVE('',#3704,#3858,#2209,.T.);
#4841=EDGE_CURVE('',#3857,#3858,#2210,.T.);
#4842=EDGE_CURVE('',#3859,#3703,#2211,.T.);
#4843=EDGE_CURVE('',#3858,#3859,#2212,.T.);
#4844=EDGE_CURVE('',#3860,#3861,#2213,.T.);
#4845=EDGE_CURVE('',#3861,#3862,#2214,.T.);
#4846=EDGE_CURVE('',#3862,#3863,#2215,.T.);
#4847=EDGE_CURVE('',#3863,#3864,#2216,.T.);
#4848=EDGE_CURVE('',#3864,#3865,#2217,.T.);
#4849=EDGE_CURVE('',#3865,#3854,#2218,.T.);
#4850=EDGE_CURVE('',#3851,#3866,#2219,.T.);
#4851=EDGE_CURVE('',#3866,#3867,#2220,.T.);
#4852=EDGE_CURVE('',#3867,#3868,#2221,.T.);
#4853=EDGE_CURVE('',#3868,#3869,#2222,.T.);
#4854=EDGE_CURVE('',#3869,#3870,#2223,.T.);
#4855=EDGE_CURVE('',#3870,#3860,#2224,.T.);
#4856=EDGE_CURVE('',#3862,#3607,#2225,.T.);
#4857=EDGE_CURVE('',#3608,#3861,#2226,.T.);
#4858=EDGE_CURVE('',#3863,#3606,#2227,.T.);
#4859=EDGE_CURVE('',#3864,#3605,#2228,.T.);
#4860=EDGE_CURVE('',#3865,#3604,#2229,.T.);
#4861=EDGE_CURVE('',#3871,#3850,#2230,.T.);
#4862=EDGE_CURVE('',#3866,#3871,#2231,.T.);
#4863=EDGE_CURVE('',#3872,#3871,#2232,.T.);
#4864=EDGE_CURVE('',#3867,#3872,#2233,.T.);
#4865=EDGE_CURVE('',#3873,#3872,#2234,.T.);
#4866=EDGE_CURVE('',#3868,#3873,#2235,.T.);
#4867=EDGE_CURVE('',#3874,#3873,#2236,.T.);
#4868=EDGE_CURVE('',#3869,#3874,#2237,.T.);
#4869=EDGE_CURVE('',#3875,#3874,#2238,.T.);
#4870=EDGE_CURVE('',#3870,#3875,#2239,.T.);
#4871=EDGE_CURVE('',#3876,#3875,#2240,.T.);
#4872=EDGE_CURVE('',#3860,#3876,#2241,.T.);
#4873=EDGE_CURVE('',#3859,#3876,#2242,.T.);
#6033=ORIENTED_EDGE('',*,*,#4460,.F.);
#6034=ORIENTED_EDGE('',*,*,#4461,.F.);
#6035=ORIENTED_EDGE('',*,*,#4462,.F.);
#6036=ORIENTED_EDGE('',*,*,#4463,.F.);
#6037=ORIENTED_EDGE('',*,*,#4464,.F.);
#6038=ORIENTED_EDGE('',*,*,#4465,.F.);
#6039=ORIENTED_EDGE('',*,*,#4466,.F.);
#6040=ORIENTED_EDGE('',*,*,#4467,.F.);
#6041=ORIENTED_EDGE('',*,*,#4468,.T.);
#6042=ORIENTED_EDGE('',*,*,#4469,.F.);
#6043=ORIENTED_EDGE('',*,*,#4470,.F.);
#6044=ORIENTED_EDGE('',*,*,#4471,.F.);
#6045=ORIENTED_EDGE('',*,*,#4472,.F.);
#6046=ORIENTED_EDGE('',*,*,#4473,.F.);
#6047=ORIENTED_EDGE('',*,*,#4474,.F.);
#6048=ORIENTED_EDGE('',*,*,#4475,.F.);
#6049=ORIENTED_EDGE('',*,*,#4476,.F.);
#6050=ORIENTED_EDGE('',*,*,#4477,.T.);
#6051=ORIENTED_EDGE('',*,*,#4478,.F.);
#6052=ORIENTED_EDGE('',*,*,#4479,.F.);
#6053=ORIENTED_EDGE('',*,*,#4480,.F.);
#6054=ORIENTED_EDGE('',*,*,#4481,.F.);
#6055=ORIENTED_EDGE('',*,*,#4482,.F.);
#6056=ORIENTED_EDGE('',*,*,#4483,.F.);
#6057=ORIENTED_EDGE('',*,*,#4484,.F.);
#6058=ORIENTED_EDGE('',*,*,#4485,.F.);
#6059=ORIENTED_EDGE('',*,*,#4486,.T.);
#6060=ORIENTED_EDGE('',*,*,#4487,.F.);
#6061=ORIENTED_EDGE('',*,*,#4488,.F.);
#6062=ORIENTED_EDGE('',*,*,#4489,.F.);
#6063=ORIENTED_EDGE('',*,*,#4490,.F.);
#6064=ORIENTED_EDGE('',*,*,#4491,.F.);
#6065=ORIENTED_EDGE('',*,*,#4492,.F.);
#6066=ORIENTED_EDGE('',*,*,#4493,.F.);
#6067=ORIENTED_EDGE('',*,*,#4494,.F.);
#6068=ORIENTED_EDGE('',*,*,#4495,.T.);
#6069=ORIENTED_EDGE('',*,*,#4496,.F.);
#6070=ORIENTED_EDGE('',*,*,#4497,.F.);
#6071=ORIENTED_EDGE('',*,*,#4498,.F.);
#6072=ORIENTED_EDGE('',*,*,#4499,.F.);
#6073=ORIENTED_EDGE('',*,*,#4500,.F.);
#6074=ORIENTED_EDGE('',*,*,#4501,.F.);
#6075=ORIENTED_EDGE('',*,*,#4502,.F.);
#6076=ORIENTED_EDGE('',*,*,#4503,.F.);
#6077=ORIENTED_EDGE('',*,*,#4504,.T.);
#6078=ORIENTED_EDGE('',*,*,#4505,.F.);
#6079=ORIENTED_EDGE('',*,*,#4506,.F.);
#6080=ORIENTED_EDGE('',*,*,#4507,.F.);
#6081=ORIENTED_EDGE('',*,*,#4508,.F.);
#6082=ORIENTED_EDGE('',*,*,#4509,.F.);
#6083=ORIENTED_EDGE('',*,*,#4510,.F.);
#6084=ORIENTED_EDGE('',*,*,#4511,.F.);
#6085=ORIENTED_EDGE('',*,*,#4512,.F.);
#6086=ORIENTED_EDGE('',*,*,#4513,.T.);
#6087=ORIENTED_EDGE('',*,*,#4514,.F.);
#6088=ORIENTED_EDGE('',*,*,#4515,.F.);
#6089=ORIENTED_EDGE('',*,*,#4516,.F.);
#6090=ORIENTED_EDGE('',*,*,#4504,.F.);
#6091=ORIENTED_EDGE('',*,*,#4517,.F.);
#6092=ORIENTED_EDGE('',*,*,#4518,.F.);
#6093=ORIENTED_EDGE('',*,*,#4519,.F.);
#6094=ORIENTED_EDGE('',*,*,#4468,.F.);
#6095=ORIENTED_EDGE('',*,*,#4520,.F.);
#6096=ORIENTED_EDGE('',*,*,#4521,.F.);
#6097=ORIENTED_EDGE('',*,*,#4522,.F.);
#6098=ORIENTED_EDGE('',*,*,#4486,.F.);
#6099=ORIENTED_EDGE('',*,*,#4523,.F.);
#6100=ORIENTED_EDGE('',*,*,#4495,.F.);
#6101=ORIENTED_EDGE('',*,*,#4524,.F.);
#6102=ORIENTED_EDGE('',*,*,#4525,.F.);
#6103=ORIENTED_EDGE('',*,*,#4526,.F.);
#6104=ORIENTED_EDGE('',*,*,#4477,.F.);
#6105=ORIENTED_EDGE('',*,*,#4527,.F.);
#6106=ORIENTED_EDGE('',*,*,#4528,.F.);
#6107=ORIENTED_EDGE('',*,*,#4529,.F.);
#6108=ORIENTED_EDGE('',*,*,#4513,.F.);
#6109=ORIENTED_EDGE('',*,*,#4530,.F.);
#6110=ORIENTED_EDGE('',*,*,#4531,.F.);
#6111=ORIENTED_EDGE('',*,*,#4532,.F.);
#6112=ORIENTED_EDGE('',*,*,#4531,.T.);
#6113=ORIENTED_EDGE('',*,*,#4533,.F.);
#6114=ORIENTED_EDGE('',*,*,#4534,.F.);
#6115=ORIENTED_EDGE('',*,*,#4535,.F.);
#6116=ORIENTED_EDGE('',*,*,#4536,.F.);
#6117=ORIENTED_EDGE('',*,*,#4537,.F.);
#6118=ORIENTED_EDGE('',*,*,#4538,.F.);
#6119=ORIENTED_EDGE('',*,*,#4539,.F.);
#6120=ORIENTED_EDGE('',*,*,#4540,.F.);
#6121=ORIENTED_EDGE('',*,*,#4515,.T.);
#6122=ORIENTED_EDGE('',*,*,#4541,.F.);
#6123=ORIENTED_EDGE('',*,*,#4542,.F.);
#6124=ORIENTED_EDGE('',*,*,#4543,.F.);
#6125=ORIENTED_EDGE('',*,*,#4544,.F.);
#6126=ORIENTED_EDGE('',*,*,#4545,.F.);
#6127=ORIENTED_EDGE('',*,*,#4546,.F.);
#6128=ORIENTED_EDGE('',*,*,#4547,.F.);
#6129=ORIENTED_EDGE('',*,*,#4548,.F.);
#6130=ORIENTED_EDGE('',*,*,#4525,.T.);
#6131=ORIENTED_EDGE('',*,*,#4549,.F.);
#6132=ORIENTED_EDGE('',*,*,#4550,.F.);
#6133=ORIENTED_EDGE('',*,*,#4551,.F.);
#6134=ORIENTED_EDGE('',*,*,#4552,.F.);
#6135=ORIENTED_EDGE('',*,*,#4553,.F.);
#6136=ORIENTED_EDGE('',*,*,#4554,.F.);
#6137=ORIENTED_EDGE('',*,*,#4555,.F.);
#6138=ORIENTED_EDGE('',*,*,#4556,.F.);
#6139=ORIENTED_EDGE('',*,*,#4521,.T.);
#6140=ORIENTED_EDGE('',*,*,#4557,.F.);
#6141=ORIENTED_EDGE('',*,*,#4558,.F.);
#6142=ORIENTED_EDGE('',*,*,#4559,.F.);
#6143=ORIENTED_EDGE('',*,*,#4560,.F.);
#6144=ORIENTED_EDGE('',*,*,#4561,.F.);
#6145=ORIENTED_EDGE('',*,*,#4562,.F.);
#6146=ORIENTED_EDGE('',*,*,#4563,.F.);
#6147=ORIENTED_EDGE('',*,*,#4564,.F.);
#6148=ORIENTED_EDGE('',*,*,#4528,.T.);
#6149=ORIENTED_EDGE('',*,*,#4565,.F.);
#6150=ORIENTED_EDGE('',*,*,#4566,.F.);
#6151=ORIENTED_EDGE('',*,*,#4567,.F.);
#6152=ORIENTED_EDGE('',*,*,#4568,.F.);
#6153=ORIENTED_EDGE('',*,*,#4569,.F.);
#6154=ORIENTED_EDGE('',*,*,#4570,.F.);
#6155=ORIENTED_EDGE('',*,*,#4571,.F.);
#6156=ORIENTED_EDGE('',*,*,#4572,.F.);
#6157=ORIENTED_EDGE('',*,*,#4518,.T.);
#6158=ORIENTED_EDGE('',*,*,#4573,.F.);
#6159=ORIENTED_EDGE('',*,*,#4574,.F.);
#6160=ORIENTED_EDGE('',*,*,#4575,.F.);
#6161=ORIENTED_EDGE('',*,*,#4576,.F.);
#6162=ORIENTED_EDGE('',*,*,#4577,.F.);
#6163=ORIENTED_EDGE('',*,*,#4578,.F.);
#6164=ORIENTED_EDGE('',*,*,#4579,.F.);
#6165=ORIENTED_EDGE('',*,*,#4505,.T.);
#6166=ORIENTED_EDGE('',*,*,#4516,.T.);
#6167=ORIENTED_EDGE('',*,*,#4540,.T.);
#6168=ORIENTED_EDGE('',*,*,#4580,.T.);
#6169=ORIENTED_EDGE('',*,*,#4581,.F.);
#6170=ORIENTED_EDGE('',*,*,#4582,.F.);
#6171=ORIENTED_EDGE('',*,*,#4583,.F.);
#6172=ORIENTED_EDGE('',*,*,#4584,.T.);
#6173=ORIENTED_EDGE('',*,*,#4539,.T.);
#6174=ORIENTED_EDGE('',*,*,#4585,.T.);
#6175=ORIENTED_EDGE('',*,*,#4586,.F.);
#6176=ORIENTED_EDGE('',*,*,#4580,.F.);
#6177=ORIENTED_EDGE('',*,*,#4506,.T.);
#6178=ORIENTED_EDGE('',*,*,#4584,.F.);
#6179=ORIENTED_EDGE('',*,*,#4587,.F.);
#6180=ORIENTED_EDGE('',*,*,#4588,.T.);
#6181=ORIENTED_EDGE('',*,*,#4538,.T.);
#6182=ORIENTED_EDGE('',*,*,#4589,.T.);
#6183=ORIENTED_EDGE('',*,*,#4590,.F.);
#6184=ORIENTED_EDGE('',*,*,#4585,.F.);
#6185=ORIENTED_EDGE('',*,*,#4537,.T.);
#6186=ORIENTED_EDGE('',*,*,#4591,.T.);
#6187=ORIENTED_EDGE('',*,*,#4592,.F.);
#6188=ORIENTED_EDGE('',*,*,#4589,.F.);
#6189=ORIENTED_EDGE('',*,*,#4536,.T.);
#6190=ORIENTED_EDGE('',*,*,#4593,.T.);
#6191=ORIENTED_EDGE('',*,*,#4594,.F.);
#6192=ORIENTED_EDGE('',*,*,#4591,.F.);
#6193=ORIENTED_EDGE('',*,*,#4535,.T.);
#6194=ORIENTED_EDGE('',*,*,#4595,.T.);
#6195=ORIENTED_EDGE('',*,*,#4596,.F.);
#6196=ORIENTED_EDGE('',*,*,#4593,.F.);
#6197=ORIENTED_EDGE('',*,*,#4534,.T.);
#6198=ORIENTED_EDGE('',*,*,#4597,.F.);
#6199=ORIENTED_EDGE('',*,*,#4598,.F.);
#6200=ORIENTED_EDGE('',*,*,#4595,.F.);
#6201=ORIENTED_EDGE('',*,*,#4599,.T.);
#6202=ORIENTED_EDGE('',*,*,#4600,.T.);
#6203=ORIENTED_EDGE('',*,*,#4601,.T.);
#6204=ORIENTED_EDGE('',*,*,#4602,.T.);
#6205=ORIENTED_EDGE('',*,*,#4603,.T.);
#6206=ORIENTED_EDGE('',*,*,#4604,.T.);
#6207=ORIENTED_EDGE('',*,*,#4587,.T.);
#6208=ORIENTED_EDGE('',*,*,#4583,.T.);
#6209=ORIENTED_EDGE('',*,*,#4605,.T.);
#6210=ORIENTED_EDGE('',*,*,#4606,.T.);
#6211=ORIENTED_EDGE('',*,*,#4607,.T.);
#6212=ORIENTED_EDGE('',*,*,#4608,.T.);
#6213=ORIENTED_EDGE('',*,*,#4609,.T.);
#6214=ORIENTED_EDGE('',*,*,#4610,.T.);
#6215=ORIENTED_EDGE('',*,*,#4511,.T.);
#6216=ORIENTED_EDGE('',*,*,#4611,.F.);
#6217=ORIENTED_EDGE('',*,*,#4600,.F.);
#6218=ORIENTED_EDGE('',*,*,#4612,.F.);
#6219=ORIENTED_EDGE('',*,*,#4510,.T.);
#6220=ORIENTED_EDGE('',*,*,#4613,.F.);
#6221=ORIENTED_EDGE('',*,*,#4601,.F.);
#6222=ORIENTED_EDGE('',*,*,#4611,.T.);
#6223=ORIENTED_EDGE('',*,*,#4509,.T.);
#6224=ORIENTED_EDGE('',*,*,#4614,.F.);
#6225=ORIENTED_EDGE('',*,*,#4602,.F.);
#6226=ORIENTED_EDGE('',*,*,#4613,.T.);
#6227=ORIENTED_EDGE('',*,*,#4508,.T.);
#6228=ORIENTED_EDGE('',*,*,#4615,.F.);
#6229=ORIENTED_EDGE('',*,*,#4603,.F.);
#6230=ORIENTED_EDGE('',*,*,#4614,.T.);
#6231=ORIENTED_EDGE('',*,*,#4507,.T.);
#6232=ORIENTED_EDGE('',*,*,#4588,.F.);
#6233=ORIENTED_EDGE('',*,*,#4604,.F.);
#6234=ORIENTED_EDGE('',*,*,#4615,.T.);
#6235=ORIENTED_EDGE('',*,*,#4582,.T.);
#6236=ORIENTED_EDGE('',*,*,#4616,.F.);
#6237=ORIENTED_EDGE('',*,*,#4617,.F.);
#6238=ORIENTED_EDGE('',*,*,#4605,.F.);
#6239=ORIENTED_EDGE('',*,*,#4617,.T.);
#6240=ORIENTED_EDGE('',*,*,#4618,.F.);
#6241=ORIENTED_EDGE('',*,*,#4619,.F.);
#6242=ORIENTED_EDGE('',*,*,#4606,.F.);
#6243=ORIENTED_EDGE('',*,*,#4619,.T.);
#6244=ORIENTED_EDGE('',*,*,#4620,.F.);
#6245=ORIENTED_EDGE('',*,*,#4621,.F.);
#6246=ORIENTED_EDGE('',*,*,#4607,.F.);
#6247=ORIENTED_EDGE('',*,*,#4621,.T.);
#6248=ORIENTED_EDGE('',*,*,#4622,.F.);
#6249=ORIENTED_EDGE('',*,*,#4623,.F.);
#6250=ORIENTED_EDGE('',*,*,#4608,.F.);
#6251=ORIENTED_EDGE('',*,*,#4623,.T.);
#6252=ORIENTED_EDGE('',*,*,#4624,.F.);
#6253=ORIENTED_EDGE('',*,*,#4625,.F.);
#6254=ORIENTED_EDGE('',*,*,#4609,.F.);
#6255=ORIENTED_EDGE('',*,*,#4625,.T.);
#6256=ORIENTED_EDGE('',*,*,#4626,.F.);
#6257=ORIENTED_EDGE('',*,*,#4627,.F.);
#6258=ORIENTED_EDGE('',*,*,#4610,.F.);
#6259=ORIENTED_EDGE('',*,*,#4512,.T.);
#6260=ORIENTED_EDGE('',*,*,#4612,.T.);
#6261=ORIENTED_EDGE('',*,*,#4599,.F.);
#6262=ORIENTED_EDGE('',*,*,#4627,.T.);
#6263=ORIENTED_EDGE('',*,*,#4628,.F.);
#6264=ORIENTED_EDGE('',*,*,#4597,.T.);
#6265=ORIENTED_EDGE('',*,*,#4533,.T.);
#6266=ORIENTED_EDGE('',*,*,#4530,.T.);
#6267=ORIENTED_EDGE('',*,*,#4628,.T.);
#6268=ORIENTED_EDGE('',*,*,#4626,.T.);
#6269=ORIENTED_EDGE('',*,*,#4624,.T.);
#6270=ORIENTED_EDGE('',*,*,#4622,.T.);
#6271=ORIENTED_EDGE('',*,*,#4620,.T.);
#6272=ORIENTED_EDGE('',*,*,#4618,.T.);
#6273=ORIENTED_EDGE('',*,*,#4616,.T.);
#6274=ORIENTED_EDGE('',*,*,#4581,.T.);
#6275=ORIENTED_EDGE('',*,*,#4586,.T.);
#6276=ORIENTED_EDGE('',*,*,#4590,.T.);
#6277=ORIENTED_EDGE('',*,*,#4592,.T.);
#6278=ORIENTED_EDGE('',*,*,#4594,.T.);
#6279=ORIENTED_EDGE('',*,*,#4596,.T.);
#6280=ORIENTED_EDGE('',*,*,#4598,.T.);
#6281=ORIENTED_EDGE('',*,*,#4469,.T.);
#6282=ORIENTED_EDGE('',*,*,#4519,.T.);
#6283=ORIENTED_EDGE('',*,*,#4572,.T.);
#6284=ORIENTED_EDGE('',*,*,#4629,.T.);
#6285=ORIENTED_EDGE('',*,*,#4630,.F.);
#6286=ORIENTED_EDGE('',*,*,#4631,.F.);
#6287=ORIENTED_EDGE('',*,*,#4632,.F.);
#6288=ORIENTED_EDGE('',*,*,#4633,.T.);
#6289=ORIENTED_EDGE('',*,*,#4571,.T.);
#6290=ORIENTED_EDGE('',*,*,#4634,.T.);
#6291=ORIENTED_EDGE('',*,*,#4635,.F.);
#6292=ORIENTED_EDGE('',*,*,#4629,.F.);
#6293=ORIENTED_EDGE('',*,*,#4470,.T.);
#6294=ORIENTED_EDGE('',*,*,#4633,.F.);
#6295=ORIENTED_EDGE('',*,*,#4636,.F.);
#6296=ORIENTED_EDGE('',*,*,#4637,.T.);
#6297=ORIENTED_EDGE('',*,*,#4570,.T.);
#6298=ORIENTED_EDGE('',*,*,#4638,.T.);
#6299=ORIENTED_EDGE('',*,*,#4639,.F.);
#6300=ORIENTED_EDGE('',*,*,#4634,.F.);
#6301=ORIENTED_EDGE('',*,*,#4569,.T.);
#6302=ORIENTED_EDGE('',*,*,#4640,.T.);
#6303=ORIENTED_EDGE('',*,*,#4641,.F.);
#6304=ORIENTED_EDGE('',*,*,#4638,.F.);
#6305=ORIENTED_EDGE('',*,*,#4568,.T.);
#6306=ORIENTED_EDGE('',*,*,#4642,.T.);
#6307=ORIENTED_EDGE('',*,*,#4643,.F.);
#6308=ORIENTED_EDGE('',*,*,#4640,.F.);
#6309=ORIENTED_EDGE('',*,*,#4567,.T.);
#6310=ORIENTED_EDGE('',*,*,#4644,.T.);
#6311=ORIENTED_EDGE('',*,*,#4645,.F.);
#6312=ORIENTED_EDGE('',*,*,#4642,.F.);
#6313=ORIENTED_EDGE('',*,*,#4566,.T.);
#6314=ORIENTED_EDGE('',*,*,#4646,.F.);
#6315=ORIENTED_EDGE('',*,*,#4647,.F.);
#6316=ORIENTED_EDGE('',*,*,#4644,.F.);
#6317=ORIENTED_EDGE('',*,*,#4648,.T.);
#6318=ORIENTED_EDGE('',*,*,#4649,.T.);
#6319=ORIENTED_EDGE('',*,*,#4650,.T.);
#6320=ORIENTED_EDGE('',*,*,#4651,.T.);
#6321=ORIENTED_EDGE('',*,*,#4652,.T.);
#6322=ORIENTED_EDGE('',*,*,#4653,.T.);
#6323=ORIENTED_EDGE('',*,*,#4636,.T.);
#6324=ORIENTED_EDGE('',*,*,#4632,.T.);
#6325=ORIENTED_EDGE('',*,*,#4654,.T.);
#6326=ORIENTED_EDGE('',*,*,#4655,.T.);
#6327=ORIENTED_EDGE('',*,*,#4656,.T.);
#6328=ORIENTED_EDGE('',*,*,#4657,.T.);
#6329=ORIENTED_EDGE('',*,*,#4658,.T.);
#6330=ORIENTED_EDGE('',*,*,#4659,.T.);
#6331=ORIENTED_EDGE('',*,*,#4475,.T.);
#6332=ORIENTED_EDGE('',*,*,#4660,.F.);
#6333=ORIENTED_EDGE('',*,*,#4649,.F.);
#6334=ORIENTED_EDGE('',*,*,#4661,.F.);
#6335=ORIENTED_EDGE('',*,*,#4474,.T.);
#6336=ORIENTED_EDGE('',*,*,#4662,.F.);
#6337=ORIENTED_EDGE('',*,*,#4650,.F.);
#6338=ORIENTED_EDGE('',*,*,#4660,.T.);
#6339=ORIENTED_EDGE('',*,*,#4473,.T.);
#6340=ORIENTED_EDGE('',*,*,#4663,.F.);
#6341=ORIENTED_EDGE('',*,*,#4651,.F.);
#6342=ORIENTED_EDGE('',*,*,#4662,.T.);
#6343=ORIENTED_EDGE('',*,*,#4472,.T.);
#6344=ORIENTED_EDGE('',*,*,#4664,.F.);
#6345=ORIENTED_EDGE('',*,*,#4652,.F.);
#6346=ORIENTED_EDGE('',*,*,#4663,.T.);
#6347=ORIENTED_EDGE('',*,*,#4471,.T.);
#6348=ORIENTED_EDGE('',*,*,#4637,.F.);
#6349=ORIENTED_EDGE('',*,*,#4653,.F.);
#6350=ORIENTED_EDGE('',*,*,#4664,.T.);
#6351=ORIENTED_EDGE('',*,*,#4631,.T.);
#6352=ORIENTED_EDGE('',*,*,#4665,.F.);
#6353=ORIENTED_EDGE('',*,*,#4666,.F.);
#6354=ORIENTED_EDGE('',*,*,#4654,.F.);
#6355=ORIENTED_EDGE('',*,*,#4666,.T.);
#6356=ORIENTED_EDGE('',*,*,#4667,.F.);
#6357=ORIENTED_EDGE('',*,*,#4668,.F.);
#6358=ORIENTED_EDGE('',*,*,#4655,.F.);
#6359=ORIENTED_EDGE('',*,*,#4668,.T.);
#6360=ORIENTED_EDGE('',*,*,#4669,.F.);
#6361=ORIENTED_EDGE('',*,*,#4670,.F.);
#6362=ORIENTED_EDGE('',*,*,#4656,.F.);
#6363=ORIENTED_EDGE('',*,*,#4670,.T.);
#6364=ORIENTED_EDGE('',*,*,#4671,.F.);
#6365=ORIENTED_EDGE('',*,*,#4672,.F.);
#6366=ORIENTED_EDGE('',*,*,#4657,.F.);
#6367=ORIENTED_EDGE('',*,*,#4672,.T.);
#6368=ORIENTED_EDGE('',*,*,#4673,.F.);
#6369=ORIENTED_EDGE('',*,*,#4674,.F.);
#6370=ORIENTED_EDGE('',*,*,#4658,.F.);
#6371=ORIENTED_EDGE('',*,*,#4674,.T.);
#6372=ORIENTED_EDGE('',*,*,#4675,.F.);
#6373=ORIENTED_EDGE('',*,*,#4676,.F.);
#6374=ORIENTED_EDGE('',*,*,#4659,.F.);
#6375=ORIENTED_EDGE('',*,*,#4476,.T.);
#6376=ORIENTED_EDGE('',*,*,#4661,.T.);
#6377=ORIENTED_EDGE('',*,*,#4648,.F.);
#6378=ORIENTED_EDGE('',*,*,#4676,.T.);
#6379=ORIENTED_EDGE('',*,*,#4677,.F.);
#6380=ORIENTED_EDGE('',*,*,#4646,.T.);
#6381=ORIENTED_EDGE('',*,*,#4565,.T.);
#6382=ORIENTED_EDGE('',*,*,#4527,.T.);
#6383=ORIENTED_EDGE('',*,*,#4677,.T.);
#6384=ORIENTED_EDGE('',*,*,#4675,.T.);
#6385=ORIENTED_EDGE('',*,*,#4673,.T.);
#6386=ORIENTED_EDGE('',*,*,#4671,.T.);
#6387=ORIENTED_EDGE('',*,*,#4669,.T.);
#6388=ORIENTED_EDGE('',*,*,#4667,.T.);
#6389=ORIENTED_EDGE('',*,*,#4665,.T.);
#6390=ORIENTED_EDGE('',*,*,#4630,.T.);
#6391=ORIENTED_EDGE('',*,*,#4635,.T.);
#6392=ORIENTED_EDGE('',*,*,#4639,.T.);
#6393=ORIENTED_EDGE('',*,*,#4641,.T.);
#6394=ORIENTED_EDGE('',*,*,#4643,.T.);
#6395=ORIENTED_EDGE('',*,*,#4645,.T.);
#6396=ORIENTED_EDGE('',*,*,#4647,.T.);
#6397=ORIENTED_EDGE('',*,*,#4487,.T.);
#6398=ORIENTED_EDGE('',*,*,#4522,.T.);
#6399=ORIENTED_EDGE('',*,*,#4556,.T.);
#6400=ORIENTED_EDGE('',*,*,#4678,.T.);
#6401=ORIENTED_EDGE('',*,*,#4679,.F.);
#6402=ORIENTED_EDGE('',*,*,#4680,.F.);
#6403=ORIENTED_EDGE('',*,*,#4681,.F.);
#6404=ORIENTED_EDGE('',*,*,#4682,.T.);
#6405=ORIENTED_EDGE('',*,*,#4555,.T.);
#6406=ORIENTED_EDGE('',*,*,#4683,.T.);
#6407=ORIENTED_EDGE('',*,*,#4684,.F.);
#6408=ORIENTED_EDGE('',*,*,#4678,.F.);
#6409=ORIENTED_EDGE('',*,*,#4488,.T.);
#6410=ORIENTED_EDGE('',*,*,#4682,.F.);
#6411=ORIENTED_EDGE('',*,*,#4685,.F.);
#6412=ORIENTED_EDGE('',*,*,#4686,.T.);
#6413=ORIENTED_EDGE('',*,*,#4554,.T.);
#6414=ORIENTED_EDGE('',*,*,#4687,.T.);
#6415=ORIENTED_EDGE('',*,*,#4688,.F.);
#6416=ORIENTED_EDGE('',*,*,#4683,.F.);
#6417=ORIENTED_EDGE('',*,*,#4553,.T.);
#6418=ORIENTED_EDGE('',*,*,#4689,.T.);
#6419=ORIENTED_EDGE('',*,*,#4690,.F.);
#6420=ORIENTED_EDGE('',*,*,#4687,.F.);
#6421=ORIENTED_EDGE('',*,*,#4552,.T.);
#6422=ORIENTED_EDGE('',*,*,#4691,.T.);
#6423=ORIENTED_EDGE('',*,*,#4692,.F.);
#6424=ORIENTED_EDGE('',*,*,#4689,.F.);
#6425=ORIENTED_EDGE('',*,*,#4551,.T.);
#6426=ORIENTED_EDGE('',*,*,#4693,.T.);
#6427=ORIENTED_EDGE('',*,*,#4694,.F.);
#6428=ORIENTED_EDGE('',*,*,#4691,.F.);
#6429=ORIENTED_EDGE('',*,*,#4550,.T.);
#6430=ORIENTED_EDGE('',*,*,#4695,.F.);
#6431=ORIENTED_EDGE('',*,*,#4696,.F.);
#6432=ORIENTED_EDGE('',*,*,#4693,.F.);
#6433=ORIENTED_EDGE('',*,*,#4697,.T.);
#6434=ORIENTED_EDGE('',*,*,#4698,.T.);
#6435=ORIENTED_EDGE('',*,*,#4699,.T.);
#6436=ORIENTED_EDGE('',*,*,#4700,.T.);
#6437=ORIENTED_EDGE('',*,*,#4701,.T.);
#6438=ORIENTED_EDGE('',*,*,#4702,.T.);
#6439=ORIENTED_EDGE('',*,*,#4685,.T.);
#6440=ORIENTED_EDGE('',*,*,#4681,.T.);
#6441=ORIENTED_EDGE('',*,*,#4703,.T.);
#6442=ORIENTED_EDGE('',*,*,#4704,.T.);
#6443=ORIENTED_EDGE('',*,*,#4705,.T.);
#6444=ORIENTED_EDGE('',*,*,#4706,.T.);
#6445=ORIENTED_EDGE('',*,*,#4707,.T.);
#6446=ORIENTED_EDGE('',*,*,#4708,.T.);
#6447=ORIENTED_EDGE('',*,*,#4493,.T.);
#6448=ORIENTED_EDGE('',*,*,#4709,.F.);
#6449=ORIENTED_EDGE('',*,*,#4698,.F.);
#6450=ORIENTED_EDGE('',*,*,#4710,.F.);
#6451=ORIENTED_EDGE('',*,*,#4492,.T.);
#6452=ORIENTED_EDGE('',*,*,#4711,.F.);
#6453=ORIENTED_EDGE('',*,*,#4699,.F.);
#6454=ORIENTED_EDGE('',*,*,#4709,.T.);
#6455=ORIENTED_EDGE('',*,*,#4491,.T.);
#6456=ORIENTED_EDGE('',*,*,#4712,.F.);
#6457=ORIENTED_EDGE('',*,*,#4700,.F.);
#6458=ORIENTED_EDGE('',*,*,#4711,.T.);
#6459=ORIENTED_EDGE('',*,*,#4490,.T.);
#6460=ORIENTED_EDGE('',*,*,#4713,.F.);
#6461=ORIENTED_EDGE('',*,*,#4701,.F.);
#6462=ORIENTED_EDGE('',*,*,#4712,.T.);
#6463=ORIENTED_EDGE('',*,*,#4489,.T.);
#6464=ORIENTED_EDGE('',*,*,#4686,.F.);
#6465=ORIENTED_EDGE('',*,*,#4702,.F.);
#6466=ORIENTED_EDGE('',*,*,#4713,.T.);
#6467=ORIENTED_EDGE('',*,*,#4680,.T.);
#6468=ORIENTED_EDGE('',*,*,#4714,.F.);
#6469=ORIENTED_EDGE('',*,*,#4715,.F.);
#6470=ORIENTED_EDGE('',*,*,#4703,.F.);
#6471=ORIENTED_EDGE('',*,*,#4715,.T.);
#6472=ORIENTED_EDGE('',*,*,#4716,.F.);
#6473=ORIENTED_EDGE('',*,*,#4717,.F.);
#6474=ORIENTED_EDGE('',*,*,#4704,.F.);
#6475=ORIENTED_EDGE('',*,*,#4717,.T.);
#6476=ORIENTED_EDGE('',*,*,#4718,.F.);
#6477=ORIENTED_EDGE('',*,*,#4719,.F.);
#6478=ORIENTED_EDGE('',*,*,#4705,.F.);
#6479=ORIENTED_EDGE('',*,*,#4719,.T.);
#6480=ORIENTED_EDGE('',*,*,#4720,.F.);
#6481=ORIENTED_EDGE('',*,*,#4721,.F.);
#6482=ORIENTED_EDGE('',*,*,#4706,.F.);
#6483=ORIENTED_EDGE('',*,*,#4721,.T.);
#6484=ORIENTED_EDGE('',*,*,#4722,.F.);
#6485=ORIENTED_EDGE('',*,*,#4723,.F.);
#6486=ORIENTED_EDGE('',*,*,#4707,.F.);
#6487=ORIENTED_EDGE('',*,*,#4723,.T.);
#6488=ORIENTED_EDGE('',*,*,#4724,.F.);
#6489=ORIENTED_EDGE('',*,*,#4725,.F.);
#6490=ORIENTED_EDGE('',*,*,#4708,.F.);
#6491=ORIENTED_EDGE('',*,*,#4494,.T.);
#6492=ORIENTED_EDGE('',*,*,#4710,.T.);
#6493=ORIENTED_EDGE('',*,*,#4697,.F.);
#6494=ORIENTED_EDGE('',*,*,#4725,.T.);
#6495=ORIENTED_EDGE('',*,*,#4726,.F.);
#6496=ORIENTED_EDGE('',*,*,#4695,.T.);
#6497=ORIENTED_EDGE('',*,*,#4549,.T.);
#6498=ORIENTED_EDGE('',*,*,#4524,.T.);
#6499=ORIENTED_EDGE('',*,*,#4726,.T.);
#6500=ORIENTED_EDGE('',*,*,#4724,.T.);
#6501=ORIENTED_EDGE('',*,*,#4722,.T.);
#6502=ORIENTED_EDGE('',*,*,#4720,.T.);
#6503=ORIENTED_EDGE('',*,*,#4718,.T.);
#6504=ORIENTED_EDGE('',*,*,#4716,.T.);
#6505=ORIENTED_EDGE('',*,*,#4714,.T.);
#6506=ORIENTED_EDGE('',*,*,#4679,.T.);
#6507=ORIENTED_EDGE('',*,*,#4684,.T.);
#6508=ORIENTED_EDGE('',*,*,#4688,.T.);
#6509=ORIENTED_EDGE('',*,*,#4690,.T.);
#6510=ORIENTED_EDGE('',*,*,#4692,.T.);
#6511=ORIENTED_EDGE('',*,*,#4694,.T.);
#6512=ORIENTED_EDGE('',*,*,#4696,.T.);
#6513=ORIENTED_EDGE('',*,*,#4496,.T.);
#6514=ORIENTED_EDGE('',*,*,#4523,.T.);
#6515=ORIENTED_EDGE('',*,*,#4548,.T.);
#6516=ORIENTED_EDGE('',*,*,#4727,.T.);
#6517=ORIENTED_EDGE('',*,*,#4728,.F.);
#6518=ORIENTED_EDGE('',*,*,#4729,.F.);
#6519=ORIENTED_EDGE('',*,*,#4730,.F.);
#6520=ORIENTED_EDGE('',*,*,#4731,.T.);
#6521=ORIENTED_EDGE('',*,*,#4547,.T.);
#6522=ORIENTED_EDGE('',*,*,#4732,.T.);
#6523=ORIENTED_EDGE('',*,*,#4733,.F.);
#6524=ORIENTED_EDGE('',*,*,#4727,.F.);
#6525=ORIENTED_EDGE('',*,*,#4497,.T.);
#6526=ORIENTED_EDGE('',*,*,#4731,.F.);
#6527=ORIENTED_EDGE('',*,*,#4734,.F.);
#6528=ORIENTED_EDGE('',*,*,#4735,.T.);
#6529=ORIENTED_EDGE('',*,*,#4546,.T.);
#6530=ORIENTED_EDGE('',*,*,#4736,.T.);
#6531=ORIENTED_EDGE('',*,*,#4737,.F.);
#6532=ORIENTED_EDGE('',*,*,#4732,.F.);
#6533=ORIENTED_EDGE('',*,*,#4545,.T.);
#6534=ORIENTED_EDGE('',*,*,#4738,.T.);
#6535=ORIENTED_EDGE('',*,*,#4739,.F.);
#6536=ORIENTED_EDGE('',*,*,#4736,.F.);
#6537=ORIENTED_EDGE('',*,*,#4544,.T.);
#6538=ORIENTED_EDGE('',*,*,#4740,.T.);
#6539=ORIENTED_EDGE('',*,*,#4741,.F.);
#6540=ORIENTED_EDGE('',*,*,#4738,.F.);
#6541=ORIENTED_EDGE('',*,*,#4543,.T.);
#6542=ORIENTED_EDGE('',*,*,#4742,.T.);
#6543=ORIENTED_EDGE('',*,*,#4743,.F.);
#6544=ORIENTED_EDGE('',*,*,#4740,.F.);
#6545=ORIENTED_EDGE('',*,*,#4542,.T.);
#6546=ORIENTED_EDGE('',*,*,#4744,.F.);
#6547=ORIENTED_EDGE('',*,*,#4745,.F.);
#6548=ORIENTED_EDGE('',*,*,#4742,.F.);
#6549=ORIENTED_EDGE('',*,*,#4746,.T.);
#6550=ORIENTED_EDGE('',*,*,#4747,.T.);
#6551=ORIENTED_EDGE('',*,*,#4748,.T.);
#6552=ORIENTED_EDGE('',*,*,#4749,.T.);
#6553=ORIENTED_EDGE('',*,*,#4750,.T.);
#6554=ORIENTED_EDGE('',*,*,#4751,.T.);
#6555=ORIENTED_EDGE('',*,*,#4734,.T.);
#6556=ORIENTED_EDGE('',*,*,#4730,.T.);
#6557=ORIENTED_EDGE('',*,*,#4752,.T.);
#6558=ORIENTED_EDGE('',*,*,#4753,.T.);
#6559=ORIENTED_EDGE('',*,*,#4754,.T.);
#6560=ORIENTED_EDGE('',*,*,#4755,.T.);
#6561=ORIENTED_EDGE('',*,*,#4756,.T.);
#6562=ORIENTED_EDGE('',*,*,#4757,.T.);
#6563=ORIENTED_EDGE('',*,*,#4502,.T.);
#6564=ORIENTED_EDGE('',*,*,#4758,.F.);
#6565=ORIENTED_EDGE('',*,*,#4747,.F.);
#6566=ORIENTED_EDGE('',*,*,#4759,.F.);
#6567=ORIENTED_EDGE('',*,*,#4501,.T.);
#6568=ORIENTED_EDGE('',*,*,#4760,.F.);
#6569=ORIENTED_EDGE('',*,*,#4748,.F.);
#6570=ORIENTED_EDGE('',*,*,#4758,.T.);
#6571=ORIENTED_EDGE('',*,*,#4500,.T.);
#6572=ORIENTED_EDGE('',*,*,#4761,.F.);
#6573=ORIENTED_EDGE('',*,*,#4749,.F.);
#6574=ORIENTED_EDGE('',*,*,#4760,.T.);
#6575=ORIENTED_EDGE('',*,*,#4499,.T.);
#6576=ORIENTED_EDGE('',*,*,#4762,.F.);
#6577=ORIENTED_EDGE('',*,*,#4750,.F.);
#6578=ORIENTED_EDGE('',*,*,#4761,.T.);
#6579=ORIENTED_EDGE('',*,*,#4498,.T.);
#6580=ORIENTED_EDGE('',*,*,#4735,.F.);
#6581=ORIENTED_EDGE('',*,*,#4751,.F.);
#6582=ORIENTED_EDGE('',*,*,#4762,.T.);
#6583=ORIENTED_EDGE('',*,*,#4729,.T.);
#6584=ORIENTED_EDGE('',*,*,#4763,.F.);
#6585=ORIENTED_EDGE('',*,*,#4764,.F.);
#6586=ORIENTED_EDGE('',*,*,#4752,.F.);
#6587=ORIENTED_EDGE('',*,*,#4764,.T.);
#6588=ORIENTED_EDGE('',*,*,#4765,.F.);
#6589=ORIENTED_EDGE('',*,*,#4766,.F.);
#6590=ORIENTED_EDGE('',*,*,#4753,.F.);
#6591=ORIENTED_EDGE('',*,*,#4766,.T.);
#6592=ORIENTED_EDGE('',*,*,#4767,.F.);
#6593=ORIENTED_EDGE('',*,*,#4768,.F.);
#6594=ORIENTED_EDGE('',*,*,#4754,.F.);
#6595=ORIENTED_EDGE('',*,*,#4768,.T.);
#6596=ORIENTED_EDGE('',*,*,#4769,.F.);
#6597=ORIENTED_EDGE('',*,*,#4770,.F.);
#6598=ORIENTED_EDGE('',*,*,#4755,.F.);
#6599=ORIENTED_EDGE('',*,*,#4770,.T.);
#6600=ORIENTED_EDGE('',*,*,#4771,.F.);
#6601=ORIENTED_EDGE('',*,*,#4772,.F.);
#6602=ORIENTED_EDGE('',*,*,#4756,.F.);
#6603=ORIENTED_EDGE('',*,*,#4772,.T.);
#6604=ORIENTED_EDGE('',*,*,#4773,.F.);
#6605=ORIENTED_EDGE('',*,*,#4774,.F.);
#6606=ORIENTED_EDGE('',*,*,#4757,.F.);
#6607=ORIENTED_EDGE('',*,*,#4503,.T.);
#6608=ORIENTED_EDGE('',*,*,#4759,.T.);
#6609=ORIENTED_EDGE('',*,*,#4746,.F.);
#6610=ORIENTED_EDGE('',*,*,#4774,.T.);
#6611=ORIENTED_EDGE('',*,*,#4775,.F.);
#6612=ORIENTED_EDGE('',*,*,#4744,.T.);
#6613=ORIENTED_EDGE('',*,*,#4541,.T.);
#6614=ORIENTED_EDGE('',*,*,#4514,.T.);
#6615=ORIENTED_EDGE('',*,*,#4775,.T.);
#6616=ORIENTED_EDGE('',*,*,#4773,.T.);
#6617=ORIENTED_EDGE('',*,*,#4771,.T.);
#6618=ORIENTED_EDGE('',*,*,#4769,.T.);
#6619=ORIENTED_EDGE('',*,*,#4767,.T.);
#6620=ORIENTED_EDGE('',*,*,#4765,.T.);
#6621=ORIENTED_EDGE('',*,*,#4763,.T.);
#6622=ORIENTED_EDGE('',*,*,#4728,.T.);
#6623=ORIENTED_EDGE('',*,*,#4733,.T.);
#6624=ORIENTED_EDGE('',*,*,#4737,.T.);
#6625=ORIENTED_EDGE('',*,*,#4739,.T.);
#6626=ORIENTED_EDGE('',*,*,#4741,.T.);
#6627=ORIENTED_EDGE('',*,*,#4743,.T.);
#6628=ORIENTED_EDGE('',*,*,#4745,.T.);
#6629=ORIENTED_EDGE('',*,*,#4478,.T.);
#6630=ORIENTED_EDGE('',*,*,#4526,.T.);
#6631=ORIENTED_EDGE('',*,*,#4564,.T.);
#6632=ORIENTED_EDGE('',*,*,#4776,.T.);
#6633=ORIENTED_EDGE('',*,*,#4777,.F.);
#6634=ORIENTED_EDGE('',*,*,#4778,.F.);
#6635=ORIENTED_EDGE('',*,*,#4779,.F.);
#6636=ORIENTED_EDGE('',*,*,#4780,.T.);
#6637=ORIENTED_EDGE('',*,*,#4563,.T.);
#6638=ORIENTED_EDGE('',*,*,#4781,.T.);
#6639=ORIENTED_EDGE('',*,*,#4782,.F.);
#6640=ORIENTED_EDGE('',*,*,#4776,.F.);
#6641=ORIENTED_EDGE('',*,*,#4479,.T.);
#6642=ORIENTED_EDGE('',*,*,#4780,.F.);
#6643=ORIENTED_EDGE('',*,*,#4783,.F.);
#6644=ORIENTED_EDGE('',*,*,#4784,.T.);
#6645=ORIENTED_EDGE('',*,*,#4562,.T.);
#6646=ORIENTED_EDGE('',*,*,#4785,.T.);
#6647=ORIENTED_EDGE('',*,*,#4786,.F.);
#6648=ORIENTED_EDGE('',*,*,#4781,.F.);
#6649=ORIENTED_EDGE('',*,*,#4561,.T.);
#6650=ORIENTED_EDGE('',*,*,#4787,.T.);
#6651=ORIENTED_EDGE('',*,*,#4788,.F.);
#6652=ORIENTED_EDGE('',*,*,#4785,.F.);
#6653=ORIENTED_EDGE('',*,*,#4560,.T.);
#6654=ORIENTED_EDGE('',*,*,#4789,.T.);
#6655=ORIENTED_EDGE('',*,*,#4790,.F.);
#6656=ORIENTED_EDGE('',*,*,#4787,.F.);
#6657=ORIENTED_EDGE('',*,*,#4559,.T.);
#6658=ORIENTED_EDGE('',*,*,#4791,.T.);
#6659=ORIENTED_EDGE('',*,*,#4792,.F.);
#6660=ORIENTED_EDGE('',*,*,#4789,.F.);
#6661=ORIENTED_EDGE('',*,*,#4558,.T.);
#6662=ORIENTED_EDGE('',*,*,#4793,.F.);
#6663=ORIENTED_EDGE('',*,*,#4794,.F.);
#6664=ORIENTED_EDGE('',*,*,#4791,.F.);
#6665=ORIENTED_EDGE('',*,*,#4795,.T.);
#6666=ORIENTED_EDGE('',*,*,#4796,.T.);
#6667=ORIENTED_EDGE('',*,*,#4797,.T.);
#6668=ORIENTED_EDGE('',*,*,#4798,.T.);
#6669=ORIENTED_EDGE('',*,*,#4799,.T.);
#6670=ORIENTED_EDGE('',*,*,#4800,.T.);
#6671=ORIENTED_EDGE('',*,*,#4783,.T.);
#6672=ORIENTED_EDGE('',*,*,#4779,.T.);
#6673=ORIENTED_EDGE('',*,*,#4801,.T.);
#6674=ORIENTED_EDGE('',*,*,#4802,.T.);
#6675=ORIENTED_EDGE('',*,*,#4803,.T.);
#6676=ORIENTED_EDGE('',*,*,#4804,.T.);
#6677=ORIENTED_EDGE('',*,*,#4805,.T.);
#6678=ORIENTED_EDGE('',*,*,#4806,.T.);
#6679=ORIENTED_EDGE('',*,*,#4484,.T.);
#6680=ORIENTED_EDGE('',*,*,#4807,.F.);
#6681=ORIENTED_EDGE('',*,*,#4796,.F.);
#6682=ORIENTED_EDGE('',*,*,#4808,.F.);
#6683=ORIENTED_EDGE('',*,*,#4483,.T.);
#6684=ORIENTED_EDGE('',*,*,#4809,.F.);
#6685=ORIENTED_EDGE('',*,*,#4797,.F.);
#6686=ORIENTED_EDGE('',*,*,#4807,.T.);
#6687=ORIENTED_EDGE('',*,*,#4482,.T.);
#6688=ORIENTED_EDGE('',*,*,#4810,.F.);
#6689=ORIENTED_EDGE('',*,*,#4798,.F.);
#6690=ORIENTED_EDGE('',*,*,#4809,.T.);
#6691=ORIENTED_EDGE('',*,*,#4481,.T.);
#6692=ORIENTED_EDGE('',*,*,#4811,.F.);
#6693=ORIENTED_EDGE('',*,*,#4799,.F.);
#6694=ORIENTED_EDGE('',*,*,#4810,.T.);
#6695=ORIENTED_EDGE('',*,*,#4480,.T.);
#6696=ORIENTED_EDGE('',*,*,#4784,.F.);
#6697=ORIENTED_EDGE('',*,*,#4800,.F.);
#6698=ORIENTED_EDGE('',*,*,#4811,.T.);
#6699=ORIENTED_EDGE('',*,*,#4778,.T.);
#6700=ORIENTED_EDGE('',*,*,#4812,.F.);
#6701=ORIENTED_EDGE('',*,*,#4813,.F.);
#6702=ORIENTED_EDGE('',*,*,#4801,.F.);
#6703=ORIENTED_EDGE('',*,*,#4813,.T.);
#6704=ORIENTED_EDGE('',*,*,#4814,.F.);
#6705=ORIENTED_EDGE('',*,*,#4815,.F.);
#6706=ORIENTED_EDGE('',*,*,#4802,.F.);
#6707=ORIENTED_EDGE('',*,*,#4815,.T.);
#6708=ORIENTED_EDGE('',*,*,#4816,.F.);
#6709=ORIENTED_EDGE('',*,*,#4817,.F.);
#6710=ORIENTED_EDGE('',*,*,#4803,.F.);
#6711=ORIENTED_EDGE('',*,*,#4817,.T.);
#6712=ORIENTED_EDGE('',*,*,#4818,.F.);
#6713=ORIENTED_EDGE('',*,*,#4819,.F.);
#6714=ORIENTED_EDGE('',*,*,#4804,.F.);
#6715=ORIENTED_EDGE('',*,*,#4819,.T.);
#6716=ORIENTED_EDGE('',*,*,#4820,.F.);
#6717=ORIENTED_EDGE('',*,*,#4821,.F.);
#6718=ORIENTED_EDGE('',*,*,#4805,.F.);
#6719=ORIENTED_EDGE('',*,*,#4821,.T.);
#6720=ORIENTED_EDGE('',*,*,#4822,.F.);
#6721=ORIENTED_EDGE('',*,*,#4823,.F.);
#6722=ORIENTED_EDGE('',*,*,#4806,.F.);
#6723=ORIENTED_EDGE('',*,*,#4485,.T.);
#6724=ORIENTED_EDGE('',*,*,#4808,.T.);
#6725=ORIENTED_EDGE('',*,*,#4795,.F.);
#6726=ORIENTED_EDGE('',*,*,#4823,.T.);
#6727=ORIENTED_EDGE('',*,*,#4824,.F.);
#6728=ORIENTED_EDGE('',*,*,#4793,.T.);
#6729=ORIENTED_EDGE('',*,*,#4557,.T.);
#6730=ORIENTED_EDGE('',*,*,#4520,.T.);
#6731=ORIENTED_EDGE('',*,*,#4824,.T.);
#6732=ORIENTED_EDGE('',*,*,#4822,.T.);
#6733=ORIENTED_EDGE('',*,*,#4820,.T.);
#6734=ORIENTED_EDGE('',*,*,#4818,.T.);
#6735=ORIENTED_EDGE('',*,*,#4816,.T.);
#6736=ORIENTED_EDGE('',*,*,#4814,.T.);
#6737=ORIENTED_EDGE('',*,*,#4812,.T.);
#6738=ORIENTED_EDGE('',*,*,#4777,.T.);
#6739=ORIENTED_EDGE('',*,*,#4782,.T.);
#6740=ORIENTED_EDGE('',*,*,#4786,.T.);
#6741=ORIENTED_EDGE('',*,*,#4788,.T.);
#6742=ORIENTED_EDGE('',*,*,#4790,.T.);
#6743=ORIENTED_EDGE('',*,*,#4792,.T.);
#6744=ORIENTED_EDGE('',*,*,#4794,.T.);
#6745=ORIENTED_EDGE('',*,*,#4460,.T.);
#6746=ORIENTED_EDGE('',*,*,#4529,.T.);
#6747=ORIENTED_EDGE('',*,*,#4532,.T.);
#6748=ORIENTED_EDGE('',*,*,#4825,.T.);
#6749=ORIENTED_EDGE('',*,*,#4826,.F.);
#6750=ORIENTED_EDGE('',*,*,#4827,.F.);
#6751=ORIENTED_EDGE('',*,*,#4828,.F.);
#6752=ORIENTED_EDGE('',*,*,#4829,.T.);
#6753=ORIENTED_EDGE('',*,*,#4579,.T.);
#6754=ORIENTED_EDGE('',*,*,#4830,.T.);
#6755=ORIENTED_EDGE('',*,*,#4831,.F.);
#6756=ORIENTED_EDGE('',*,*,#4825,.F.);
#6757=ORIENTED_EDGE('',*,*,#4461,.T.);
#6758=ORIENTED_EDGE('',*,*,#4829,.F.);
#6759=ORIENTED_EDGE('',*,*,#4832,.F.);
#6760=ORIENTED_EDGE('',*,*,#4833,.T.);
#6761=ORIENTED_EDGE('',*,*,#4578,.T.);
#6762=ORIENTED_EDGE('',*,*,#4834,.T.);
#6763=ORIENTED_EDGE('',*,*,#4835,.F.);
#6764=ORIENTED_EDGE('',*,*,#4830,.F.);
#6765=ORIENTED_EDGE('',*,*,#4577,.T.);
#6766=ORIENTED_EDGE('',*,*,#4836,.T.);
#6767=ORIENTED_EDGE('',*,*,#4837,.F.);
#6768=ORIENTED_EDGE('',*,*,#4834,.F.);
#6769=ORIENTED_EDGE('',*,*,#4576,.T.);
#6770=ORIENTED_EDGE('',*,*,#4838,.T.);
#6771=ORIENTED_EDGE('',*,*,#4839,.F.);
#6772=ORIENTED_EDGE('',*,*,#4836,.F.);
#6773=ORIENTED_EDGE('',*,*,#4575,.T.);
#6774=ORIENTED_EDGE('',*,*,#4840,.T.);
#6775=ORIENTED_EDGE('',*,*,#4841,.F.);
#6776=ORIENTED_EDGE('',*,*,#4838,.F.);
#6777=ORIENTED_EDGE('',*,*,#4574,.T.);
#6778=ORIENTED_EDGE('',*,*,#4842,.F.);
#6779=ORIENTED_EDGE('',*,*,#4843,.F.);
#6780=ORIENTED_EDGE('',*,*,#4840,.F.);
#6781=ORIENTED_EDGE('',*,*,#4844,.T.);
#6782=ORIENTED_EDGE('',*,*,#4845,.T.);
#6783=ORIENTED_EDGE('',*,*,#4846,.T.);
#6784=ORIENTED_EDGE('',*,*,#4847,.T.);
#6785=ORIENTED_EDGE('',*,*,#4848,.T.);
#6786=ORIENTED_EDGE('',*,*,#4849,.T.);
#6787=ORIENTED_EDGE('',*,*,#4832,.T.);
#6788=ORIENTED_EDGE('',*,*,#4828,.T.);
#6789=ORIENTED_EDGE('',*,*,#4850,.T.);
#6790=ORIENTED_EDGE('',*,*,#4851,.T.);
#6791=ORIENTED_EDGE('',*,*,#4852,.T.);
#6792=ORIENTED_EDGE('',*,*,#4853,.T.);
#6793=ORIENTED_EDGE('',*,*,#4854,.T.);
#6794=ORIENTED_EDGE('',*,*,#4855,.T.);
#6795=ORIENTED_EDGE('',*,*,#4466,.T.);
#6796=ORIENTED_EDGE('',*,*,#4856,.F.);
#6797=ORIENTED_EDGE('',*,*,#4845,.F.);
#6798=ORIENTED_EDGE('',*,*,#4857,.F.);
#6799=ORIENTED_EDGE('',*,*,#4465,.T.);
#6800=ORIENTED_EDGE('',*,*,#4858,.F.);
#6801=ORIENTED_EDGE('',*,*,#4846,.F.);
#6802=ORIENTED_EDGE('',*,*,#4856,.T.);
#6803=ORIENTED_EDGE('',*,*,#4464,.T.);
#6804=ORIENTED_EDGE('',*,*,#4859,.F.);
#6805=ORIENTED_EDGE('',*,*,#4847,.F.);
#6806=ORIENTED_EDGE('',*,*,#4858,.T.);
#6807=ORIENTED_EDGE('',*,*,#4463,.T.);
#6808=ORIENTED_EDGE('',*,*,#4860,.F.);
#6809=ORIENTED_EDGE('',*,*,#4848,.F.);
#6810=ORIENTED_EDGE('',*,*,#4859,.T.);
#6811=ORIENTED_EDGE('',*,*,#4462,.T.);
#6812=ORIENTED_EDGE('',*,*,#4833,.F.);
#6813=ORIENTED_EDGE('',*,*,#4849,.F.);
#6814=ORIENTED_EDGE('',*,*,#4860,.T.);
#6815=ORIENTED_EDGE('',*,*,#4827,.T.);
#6816=ORIENTED_EDGE('',*,*,#4861,.F.);
#6817=ORIENTED_EDGE('',*,*,#4862,.F.);
#6818=ORIENTED_EDGE('',*,*,#4850,.F.);
#6819=ORIENTED_EDGE('',*,*,#4862,.T.);
#6820=ORIENTED_EDGE('',*,*,#4863,.F.);
#6821=ORIENTED_EDGE('',*,*,#4864,.F.);
#6822=ORIENTED_EDGE('',*,*,#4851,.F.);
#6823=ORIENTED_EDGE('',*,*,#4864,.T.);
#6824=ORIENTED_EDGE('',*,*,#4865,.F.);
#6825=ORIENTED_EDGE('',*,*,#4866,.F.);
#6826=ORIENTED_EDGE('',*,*,#4852,.F.);
#6827=ORIENTED_EDGE('',*,*,#4866,.T.);
#6828=ORIENTED_EDGE('',*,*,#4867,.F.);
#6829=ORIENTED_EDGE('',*,*,#4868,.F.);
#6830=ORIENTED_EDGE('',*,*,#4853,.F.);
#6831=ORIENTED_EDGE('',*,*,#4868,.T.);
#6832=ORIENTED_EDGE('',*,*,#4869,.F.);
#6833=ORIENTED_EDGE('',*,*,#4870,.F.);
#6834=ORIENTED_EDGE('',*,*,#4854,.F.);
#6835=ORIENTED_EDGE('',*,*,#4870,.T.);
#6836=ORIENTED_EDGE('',*,*,#4871,.F.);
#6837=ORIENTED_EDGE('',*,*,#4872,.F.);
#6838=ORIENTED_EDGE('',*,*,#4855,.F.);
#6839=ORIENTED_EDGE('',*,*,#4467,.T.);
#6840=ORIENTED_EDGE('',*,*,#4857,.T.);
#6841=ORIENTED_EDGE('',*,*,#4844,.F.);
#6842=ORIENTED_EDGE('',*,*,#4872,.T.);
#6843=ORIENTED_EDGE('',*,*,#4873,.F.);
#6844=ORIENTED_EDGE('',*,*,#4842,.T.);
#6845=ORIENTED_EDGE('',*,*,#4573,.T.);
#6846=ORIENTED_EDGE('',*,*,#4517,.T.);
#6847=ORIENTED_EDGE('',*,*,#4873,.T.);
#6848=ORIENTED_EDGE('',*,*,#4871,.T.);
#6849=ORIENTED_EDGE('',*,*,#4869,.T.);
#6850=ORIENTED_EDGE('',*,*,#4867,.T.);
#6851=ORIENTED_EDGE('',*,*,#4865,.T.);
#6852=ORIENTED_EDGE('',*,*,#4863,.T.);
#6853=ORIENTED_EDGE('',*,*,#4861,.T.);
#6854=ORIENTED_EDGE('',*,*,#4826,.T.);
#6855=ORIENTED_EDGE('',*,*,#4831,.T.);
#6856=ORIENTED_EDGE('',*,*,#4835,.T.);
#6857=ORIENTED_EDGE('',*,*,#4837,.T.);
#6858=ORIENTED_EDGE('',*,*,#4839,.T.);
#6859=ORIENTED_EDGE('',*,*,#4841,.T.);
#6860=ORIENTED_EDGE('',*,*,#4843,.T.);
#6937=CYLINDRICAL_SURFACE('',#7861,0.817);
#6938=CYLINDRICAL_SURFACE('',#7863,0.817);
#6939=CYLINDRICAL_SURFACE('',#7865,0.817);
#6940=CYLINDRICAL_SURFACE('',#7867,0.817);
#6941=CYLINDRICAL_SURFACE('',#7869,0.817);
#6942=CYLINDRICAL_SURFACE('',#7871,0.817);
#7195=ADVANCED_FACE('',(#804),#410,.F.);
#7196=ADVANCED_FACE('',(#805),#6937,.T.);
#7197=ADVANCED_FACE('',(#806),#6938,.T.);
#7198=ADVANCED_FACE('',(#807),#6939,.T.);
#7199=ADVANCED_FACE('',(#808),#6940,.T.);
#7200=ADVANCED_FACE('',(#809),#6941,.T.);
#7201=ADVANCED_FACE('',(#810),#6942,.T.);
#7202=ADVANCED_FACE('',(#811),#411,.T.);
#7203=ADVANCED_FACE('',(#812),#412,.T.);
#7204=ADVANCED_FACE('',(#813),#413,.T.);
#7205=ADVANCED_FACE('',(#814),#414,.T.);
#7206=ADVANCED_FACE('',(#815),#415,.T.);
#7207=ADVANCED_FACE('',(#816),#416,.T.);
#7208=ADVANCED_FACE('',(#817),#417,.T.);
#7209=ADVANCED_FACE('',(#818),#418,.T.);
#7210=ADVANCED_FACE('',(#819),#419,.T.);
#7211=ADVANCED_FACE('',(#820),#420,.T.);
#7212=ADVANCED_FACE('',(#821),#421,.T.);
#7213=ADVANCED_FACE('',(#822),#422,.T.);
#7214=ADVANCED_FACE('',(#823),#423,.T.);
#7215=ADVANCED_FACE('',(#824),#424,.T.);
#7216=ADVANCED_FACE('',(#825),#425,.T.);
#7217=ADVANCED_FACE('',(#826),#426,.T.);
#7218=ADVANCED_FACE('',(#827),#427,.T.);
#7219=ADVANCED_FACE('',(#828),#428,.T.);
#7220=ADVANCED_FACE('',(#829),#429,.T.);
#7221=ADVANCED_FACE('',(#830),#430,.T.);
#7222=ADVANCED_FACE('',(#831),#431,.T.);
#7223=ADVANCED_FACE('',(#832),#432,.T.);
#7224=ADVANCED_FACE('',(#833),#433,.T.);
#7225=ADVANCED_FACE('',(#834),#434,.T.);
#7226=ADVANCED_FACE('',(#835),#435,.T.);
#7227=ADVANCED_FACE('',(#836),#436,.T.);
#7228=ADVANCED_FACE('',(#837),#437,.T.);
#7229=ADVANCED_FACE('',(#838),#438,.T.);
#7230=ADVANCED_FACE('',(#839),#439,.T.);
#7231=ADVANCED_FACE('',(#840),#440,.T.);
#7232=ADVANCED_FACE('',(#841),#441,.T.);
#7233=ADVANCED_FACE('',(#842),#442,.T.);
#7234=ADVANCED_FACE('',(#843),#443,.T.);
#7235=ADVANCED_FACE('',(#844),#444,.T.);
#7236=ADVANCED_FACE('',(#845),#445,.T.);
#7237=ADVANCED_FACE('',(#846),#446,.T.);
#7238=ADVANCED_FACE('',(#847),#447,.T.);
#7239=ADVANCED_FACE('',(#848),#448,.T.);
#7240=ADVANCED_FACE('',(#849),#449,.T.);
#7241=ADVANCED_FACE('',(#850),#450,.T.);
#7242=ADVANCED_FACE('',(#851),#451,.T.);
#7243=ADVANCED_FACE('',(#852),#452,.T.);
#7244=ADVANCED_FACE('',(#853),#453,.T.);
#7245=ADVANCED_FACE('',(#854),#454,.T.);
#7246=ADVANCED_FACE('',(#855),#455,.T.);
#7247=ADVANCED_FACE('',(#856),#456,.T.);
#7248=ADVANCED_FACE('',(#857),#457,.T.);
#7249=ADVANCED_FACE('',(#858),#458,.T.);
#7250=ADVANCED_FACE('',(#859),#459,.T.);
#7251=ADVANCED_FACE('',(#860),#460,.T.);
#7252=ADVANCED_FACE('',(#861),#461,.T.);
#7253=ADVANCED_FACE('',(#862),#462,.T.);
#7254=ADVANCED_FACE('',(#863),#463,.T.);
#7255=ADVANCED_FACE('',(#864),#464,.T.);
#7256=ADVANCED_FACE('',(#865),#465,.T.);
#7257=ADVANCED_FACE('',(#866),#466,.T.);
#7258=ADVANCED_FACE('',(#867),#467,.T.);
#7259=ADVANCED_FACE('',(#868),#468,.T.);
#7260=ADVANCED_FACE('',(#869),#469,.T.);
#7261=ADVANCED_FACE('',(#870),#470,.T.);
#7262=ADVANCED_FACE('',(#871),#471,.T.);
#7263=ADVANCED_FACE('',(#872),#472,.T.);
#7264=ADVANCED_FACE('',(#873),#473,.T.);
#7265=ADVANCED_FACE('',(#874),#474,.T.);
#7266=ADVANCED_FACE('',(#875),#475,.T.);
#7267=ADVANCED_FACE('',(#876),#476,.T.);
#7268=ADVANCED_FACE('',(#877),#477,.T.);
#7269=ADVANCED_FACE('',(#878),#478,.T.);
#7270=ADVANCED_FACE('',(#879),#479,.T.);
#7271=ADVANCED_FACE('',(#880),#480,.T.);
#7272=ADVANCED_FACE('',(#881),#481,.T.);
#7273=ADVANCED_FACE('',(#882),#482,.T.);
#7274=ADVANCED_FACE('',(#883),#483,.T.);
#7275=ADVANCED_FACE('',(#884),#484,.T.);
#7276=ADVANCED_FACE('',(#885),#485,.T.);
#7277=ADVANCED_FACE('',(#886),#486,.T.);
#7278=ADVANCED_FACE('',(#887),#487,.T.);
#7279=ADVANCED_FACE('',(#888),#488,.T.);
#7280=ADVANCED_FACE('',(#889),#489,.T.);
#7281=ADVANCED_FACE('',(#890),#490,.T.);
#7282=ADVANCED_FACE('',(#891),#491,.T.);
#7283=ADVANCED_FACE('',(#892),#492,.T.);
#7284=ADVANCED_FACE('',(#893),#493,.T.);
#7285=ADVANCED_FACE('',(#894),#494,.T.);
#7286=ADVANCED_FACE('',(#895),#495,.T.);
#7287=ADVANCED_FACE('',(#896),#496,.T.);
#7288=ADVANCED_FACE('',(#897),#497,.T.);
#7289=ADVANCED_FACE('',(#898),#498,.T.);
#7290=ADVANCED_FACE('',(#899),#499,.T.);
#7291=ADVANCED_FACE('',(#900),#500,.T.);
#7292=ADVANCED_FACE('',(#901),#501,.T.);
#7293=ADVANCED_FACE('',(#902),#502,.T.);
#7294=ADVANCED_FACE('',(#903),#503,.T.);
#7295=ADVANCED_FACE('',(#904),#504,.T.);
#7296=ADVANCED_FACE('',(#905),#505,.T.);
#7297=ADVANCED_FACE('',(#906),#506,.T.);
#7298=ADVANCED_FACE('',(#907),#507,.T.);
#7299=ADVANCED_FACE('',(#908),#508,.T.);
#7300=ADVANCED_FACE('',(#909),#509,.T.);
#7301=ADVANCED_FACE('',(#910),#510,.T.);
#7302=ADVANCED_FACE('',(#911),#511,.T.);
#7303=ADVANCED_FACE('',(#912),#512,.T.);
#7304=ADVANCED_FACE('',(#913),#513,.T.);
#7305=ADVANCED_FACE('',(#914),#514,.T.);
#7306=ADVANCED_FACE('',(#915),#515,.T.);
#7307=ADVANCED_FACE('',(#916),#516,.T.);
#7308=ADVANCED_FACE('',(#917),#517,.T.);
#7309=ADVANCED_FACE('',(#918),#518,.T.);
#7310=ADVANCED_FACE('',(#919),#519,.T.);
#7311=ADVANCED_FACE('',(#920),#520,.T.);
#7312=ADVANCED_FACE('',(#921),#521,.T.);
#7313=ADVANCED_FACE('',(#922),#522,.T.);
#7314=ADVANCED_FACE('',(#923),#523,.T.);
#7315=ADVANCED_FACE('',(#924),#524,.T.);
#7316=ADVANCED_FACE('',(#925),#525,.T.);
#7317=ADVANCED_FACE('',(#926),#526,.T.);
#7318=ADVANCED_FACE('',(#927),#527,.T.);
#7319=ADVANCED_FACE('',(#928),#528,.T.);
#7320=ADVANCED_FACE('',(#929),#529,.T.);
#7321=ADVANCED_FACE('',(#930),#530,.T.);
#7322=ADVANCED_FACE('',(#931),#531,.T.);
#7323=ADVANCED_FACE('',(#932),#532,.T.);
#7324=ADVANCED_FACE('',(#933),#533,.T.);
#7325=ADVANCED_FACE('',(#934),#534,.T.);
#7326=ADVANCED_FACE('',(#935),#535,.T.);
#7327=ADVANCED_FACE('',(#936),#536,.T.);
#7328=ADVANCED_FACE('',(#937),#537,.T.);
#7329=ADVANCED_FACE('',(#938),#538,.T.);
#7330=ADVANCED_FACE('',(#939),#539,.T.);
#7331=ADVANCED_FACE('',(#940),#540,.T.);
#7332=ADVANCED_FACE('',(#941),#541,.T.);
#7333=ADVANCED_FACE('',(#942),#542,.T.);
#7334=ADVANCED_FACE('',(#943),#543,.T.);
#7358=CLOSED_SHELL('',(#7195,#7196,#7197,#7198,#7199,#7200,#7201,#7202,
#7203,#7204,#7205,#7206,#7207,#7208,#7209,#7210,#7211,#7212,#7213,#7214,
#7215,#7216,#7217,#7218,#7219,#7220,#7221,#7222,#7223,#7224,#7225,#7226,
#7227,#7228,#7229,#7230,#7231,#7232,#7233,#7234,#7235,#7236,#7237,#7238,
#7239,#7240,#7241,#7242,#7243,#7244,#7245,#7246,#7247,#7248,#7249,#7250,
#7251,#7252,#7253,#7254,#7255,#7256,#7257,#7258,#7259,#7260,#7261,#7262,
#7263,#7264,#7265,#7266,#7267,#7268,#7269,#7270,#7271,#7272,#7273,#7274,
#7275,#7276,#7277,#7278,#7279,#7280,#7281,#7282,#7283,#7284,#7285,#7286,
#7287,#7288,#7289,#7290,#7291,#7292,#7293,#7294,#7295,#7296,#7297,#7298,
#7299,#7300,#7301,#7302,#7303,#7304,#7305,#7306,#7307,#7308,#7309,#7310,
#7311,#7312,#7313,#7314,#7315,#7316,#7317,#7318,#7319,#7320,#7321,#7322,
#7323,#7324,#7325,#7326,#7327,#7328,#7329,#7330,#7331,#7332,#7333,#7334));
#7853=AXIS2_PLACEMENT_3D('',#11410,#9235,#9236);
#7854=AXIS2_PLACEMENT_3D('',#11411,#9237,#9238);
#7855=AXIS2_PLACEMENT_3D('',#11430,#9247,#9248);
#7856=AXIS2_PLACEMENT_3D('',#11448,#9257,#9258);
#7857=AXIS2_PLACEMENT_3D('',#11466,#9267,#9268);
#7858=AXIS2_PLACEMENT_3D('',#11484,#9277,#9278);
#7859=AXIS2_PLACEMENT_3D('',#11502,#9287,#9288);
#7860=AXIS2_PLACEMENT_3D('',#11519,#9297,#9298);
#7861=AXIS2_PLACEMENT_3D('',#11520,#9299,#9300);
#7862=AXIS2_PLACEMENT_3D('',#11524,#9302,#9303);
#7863=AXIS2_PLACEMENT_3D('',#11526,#9305,#9306);
#7864=AXIS2_PLACEMENT_3D('',#11530,#9308,#9309);
#7865=AXIS2_PLACEMENT_3D('',#11532,#9311,#9312);
#7866=AXIS2_PLACEMENT_3D('',#11536,#9314,#9315);
#7867=AXIS2_PLACEMENT_3D('',#11538,#9317,#9318);
#7868=AXIS2_PLACEMENT_3D('',#11543,#9321,#9322);
#7869=AXIS2_PLACEMENT_3D('',#11544,#9323,#9324);
#7870=AXIS2_PLACEMENT_3D('',#11549,#9327,#9328);
#7871=AXIS2_PLACEMENT_3D('',#11550,#9329,#9330);
#7872=AXIS2_PLACEMENT_3D('',#11555,#9333,#9334);
#7873=AXIS2_PLACEMENT_3D('',#11556,#9335,#9336);
#7874=AXIS2_PLACEMENT_3D('',#11647,#9385,#9386);
#7875=AXIS2_PLACEMENT_3D('',#11657,#9392,#9393);
#7876=AXIS2_PLACEMENT_3D('',#11661,#9396,#9397);
#7877=AXIS2_PLACEMENT_3D('',#11665,#9400,#9401);
#7878=AXIS2_PLACEMENT_3D('',#11669,#9404,#9405);
#7879=AXIS2_PLACEMENT_3D('',#11673,#9408,#9409);
#7880=AXIS2_PLACEMENT_3D('',#11677,#9412,#9413);
#7881=AXIS2_PLACEMENT_3D('',#11681,#9416,#9417);
#7882=AXIS2_PLACEMENT_3D('',#11685,#9420,#9421);
#7883=AXIS2_PLACEMENT_3D('',#11709,#9434,#9435);
#7884=AXIS2_PLACEMENT_3D('',#11712,#9438,#9439);
#7885=AXIS2_PLACEMENT_3D('',#11714,#9441,#9442);
#7886=AXIS2_PLACEMENT_3D('',#11716,#9444,#9445);
#7887=AXIS2_PLACEMENT_3D('',#11718,#9447,#9448);
#7888=AXIS2_PLACEMENT_3D('',#11719,#9449,#9450);
#7889=AXIS2_PLACEMENT_3D('',#11723,#9453,#9454);
#7890=AXIS2_PLACEMENT_3D('',#11727,#9457,#9458);
#7891=AXIS2_PLACEMENT_3D('',#11731,#9461,#9462);
#7892=AXIS2_PLACEMENT_3D('',#11735,#9465,#9466);
#7893=AXIS2_PLACEMENT_3D('',#11739,#9469,#9470);
#7894=AXIS2_PLACEMENT_3D('',#11743,#9473,#9474);
#7895=AXIS2_PLACEMENT_3D('',#11745,#9476,#9477);
#7896=AXIS2_PLACEMENT_3D('',#11746,#9478,#9479);
#7897=AXIS2_PLACEMENT_3D('',#11756,#9485,#9486);
#7898=AXIS2_PLACEMENT_3D('',#11760,#9489,#9490);
#7899=AXIS2_PLACEMENT_3D('',#11764,#9493,#9494);
#7900=AXIS2_PLACEMENT_3D('',#11768,#9497,#9498);
#7901=AXIS2_PLACEMENT_3D('',#11772,#9501,#9502);
#7902=AXIS2_PLACEMENT_3D('',#11776,#9505,#9506);
#7903=AXIS2_PLACEMENT_3D('',#11780,#9509,#9510);
#7904=AXIS2_PLACEMENT_3D('',#11784,#9513,#9514);
#7905=AXIS2_PLACEMENT_3D('',#11808,#9527,#9528);
#7906=AXIS2_PLACEMENT_3D('',#11811,#9531,#9532);
#7907=AXIS2_PLACEMENT_3D('',#11813,#9534,#9535);
#7908=AXIS2_PLACEMENT_3D('',#11815,#9537,#9538);
#7909=AXIS2_PLACEMENT_3D('',#11817,#9540,#9541);
#7910=AXIS2_PLACEMENT_3D('',#11818,#9542,#9543);
#7911=AXIS2_PLACEMENT_3D('',#11822,#9546,#9547);
#7912=AXIS2_PLACEMENT_3D('',#11826,#9550,#9551);
#7913=AXIS2_PLACEMENT_3D('',#11830,#9554,#9555);
#7914=AXIS2_PLACEMENT_3D('',#11834,#9558,#9559);
#7915=AXIS2_PLACEMENT_3D('',#11838,#9562,#9563);
#7916=AXIS2_PLACEMENT_3D('',#11842,#9566,#9567);
#7917=AXIS2_PLACEMENT_3D('',#11844,#9569,#9570);
#7918=AXIS2_PLACEMENT_3D('',#11845,#9571,#9572);
#7919=AXIS2_PLACEMENT_3D('',#11855,#9578,#9579);
#7920=AXIS2_PLACEMENT_3D('',#11859,#9582,#9583);
#7921=AXIS2_PLACEMENT_3D('',#11863,#9586,#9587);
#7922=AXIS2_PLACEMENT_3D('',#11867,#9590,#9591);
#7923=AXIS2_PLACEMENT_3D('',#11871,#9594,#9595);
#7924=AXIS2_PLACEMENT_3D('',#11875,#9598,#9599);
#7925=AXIS2_PLACEMENT_3D('',#11879,#9602,#9603);
#7926=AXIS2_PLACEMENT_3D('',#11883,#9606,#9607);
#7927=AXIS2_PLACEMENT_3D('',#11907,#9620,#9621);
#7928=AXIS2_PLACEMENT_3D('',#11910,#9624,#9625);
#7929=AXIS2_PLACEMENT_3D('',#11912,#9627,#9628);
#7930=AXIS2_PLACEMENT_3D('',#11914,#9630,#9631);
#7931=AXIS2_PLACEMENT_3D('',#11916,#9633,#9634);
#7932=AXIS2_PLACEMENT_3D('',#11917,#9635,#9636);
#7933=AXIS2_PLACEMENT_3D('',#11921,#9639,#9640);
#7934=AXIS2_PLACEMENT_3D('',#11925,#9643,#9644);
#7935=AXIS2_PLACEMENT_3D('',#11929,#9647,#9648);
#7936=AXIS2_PLACEMENT_3D('',#11933,#9651,#9652);
#7937=AXIS2_PLACEMENT_3D('',#11937,#9655,#9656);
#7938=AXIS2_PLACEMENT_3D('',#11941,#9659,#9660);
#7939=AXIS2_PLACEMENT_3D('',#11943,#9662,#9663);
#7940=AXIS2_PLACEMENT_3D('',#11944,#9664,#9665);
#7941=AXIS2_PLACEMENT_3D('',#11954,#9671,#9672);
#7942=AXIS2_PLACEMENT_3D('',#11958,#9675,#9676);
#7943=AXIS2_PLACEMENT_3D('',#11962,#9679,#9680);
#7944=AXIS2_PLACEMENT_3D('',#11966,#9683,#9684);
#7945=AXIS2_PLACEMENT_3D('',#11970,#9687,#9688);
#7946=AXIS2_PLACEMENT_3D('',#11974,#9691,#9692);
#7947=AXIS2_PLACEMENT_3D('',#11978,#9695,#9696);
#7948=AXIS2_PLACEMENT_3D('',#11982,#9699,#9700);
#7949=AXIS2_PLACEMENT_3D('',#12006,#9713,#9714);
#7950=AXIS2_PLACEMENT_3D('',#12009,#9717,#9718);
#7951=AXIS2_PLACEMENT_3D('',#12011,#9720,#9721);
#7952=AXIS2_PLACEMENT_3D('',#12013,#9723,#9724);
#7953=AXIS2_PLACEMENT_3D('',#12015,#9726,#9727);
#7954=AXIS2_PLACEMENT_3D('',#12016,#9728,#9729);
#7955=AXIS2_PLACEMENT_3D('',#12020,#9732,#9733);
#7956=AXIS2_PLACEMENT_3D('',#12024,#9736,#9737);
#7957=AXIS2_PLACEMENT_3D('',#12028,#9740,#9741);
#7958=AXIS2_PLACEMENT_3D('',#12032,#9744,#9745);
#7959=AXIS2_PLACEMENT_3D('',#12036,#9748,#9749);
#7960=AXIS2_PLACEMENT_3D('',#12040,#9752,#9753);
#7961=AXIS2_PLACEMENT_3D('',#12042,#9755,#9756);
#7962=AXIS2_PLACEMENT_3D('',#12043,#9757,#9758);
#7963=AXIS2_PLACEMENT_3D('',#12053,#9764,#9765);
#7964=AXIS2_PLACEMENT_3D('',#12057,#9768,#9769);
#7965=AXIS2_PLACEMENT_3D('',#12061,#9772,#9773);
#7966=AXIS2_PLACEMENT_3D('',#12065,#9776,#9777);
#7967=AXIS2_PLACEMENT_3D('',#12069,#9780,#9781);
#7968=AXIS2_PLACEMENT_3D('',#12073,#9784,#9785);
#7969=AXIS2_PLACEMENT_3D('',#12077,#9788,#9789);
#7970=AXIS2_PLACEMENT_3D('',#12081,#9792,#9793);
#7971=AXIS2_PLACEMENT_3D('',#12105,#9806,#9807);
#7972=AXIS2_PLACEMENT_3D('',#12108,#9810,#9811);
#7973=AXIS2_PLACEMENT_3D('',#12110,#9813,#9814);
#7974=AXIS2_PLACEMENT_3D('',#12112,#9816,#9817);
#7975=AXIS2_PLACEMENT_3D('',#12114,#9819,#9820);
#7976=AXIS2_PLACEMENT_3D('',#12115,#9821,#9822);
#7977=AXIS2_PLACEMENT_3D('',#12119,#9825,#9826);
#7978=AXIS2_PLACEMENT_3D('',#12123,#9829,#9830);
#7979=AXIS2_PLACEMENT_3D('',#12127,#9833,#9834);
#7980=AXIS2_PLACEMENT_3D('',#12131,#9837,#9838);
#7981=AXIS2_PLACEMENT_3D('',#12135,#9841,#9842);
#7982=AXIS2_PLACEMENT_3D('',#12139,#9845,#9846);
#7983=AXIS2_PLACEMENT_3D('',#12141,#9848,#9849);
#7984=AXIS2_PLACEMENT_3D('',#12142,#9850,#9851);
#7985=AXIS2_PLACEMENT_3D('',#12152,#9857,#9858);
#7986=AXIS2_PLACEMENT_3D('',#12156,#9861,#9862);
#7987=AXIS2_PLACEMENT_3D('',#12160,#9865,#9866);
#7988=AXIS2_PLACEMENT_3D('',#12164,#9869,#9870);
#7989=AXIS2_PLACEMENT_3D('',#12168,#9873,#9874);
#7990=AXIS2_PLACEMENT_3D('',#12172,#9877,#9878);
#7991=AXIS2_PLACEMENT_3D('',#12176,#9881,#9882);
#7992=AXIS2_PLACEMENT_3D('',#12180,#9885,#9886);
#7993=AXIS2_PLACEMENT_3D('',#12204,#9899,#9900);
#7994=AXIS2_PLACEMENT_3D('',#12207,#9903,#9904);
#7995=AXIS2_PLACEMENT_3D('',#12209,#9906,#9907);
#7996=AXIS2_PLACEMENT_3D('',#12211,#9909,#9910);
#7997=AXIS2_PLACEMENT_3D('',#12213,#9912,#9913);
#7998=AXIS2_PLACEMENT_3D('',#12214,#9914,#9915);
#7999=AXIS2_PLACEMENT_3D('',#12218,#9918,#9919);
#8000=AXIS2_PLACEMENT_3D('',#12222,#9922,#9923);
#8001=AXIS2_PLACEMENT_3D('',#12226,#9926,#9927);
#8002=AXIS2_PLACEMENT_3D('',#12230,#9930,#9931);
#8003=AXIS2_PLACEMENT_3D('',#12234,#9934,#9935);
#8004=AXIS2_PLACEMENT_3D('',#12238,#9938,#9939);
#8005=AXIS2_PLACEMENT_3D('',#12240,#9941,#9942);
#9235=DIRECTION('axis',(0.,0.,1.));
#9236=DIRECTION('refdir',(1.,0.,0.));
#9237=DIRECTION('center_axis',(0.,1.,0.));
#9238=DIRECTION('ref_axis',(0.866025403784439,0.,-0.5));
#9239=DIRECTION('',(0.121869343405147,0.,0.992546151641322));
#9240=DIRECTION('',(0.994821748296033,0.,-0.101635078182804));
#9241=DIRECTION('',(0.998134798421867,0.,-0.0610485395348574));
#9242=DIRECTION('',(0.999792698085389,0.,-0.0203607675478923));
#9243=DIRECTION('',(0.999792698085388,0.,0.0203607675478936));
#9244=DIRECTION('',(0.998134798421867,0.,0.0610485395348586));
#9245=DIRECTION('',(0.994821748296033,0.,0.101635078182805));
#9246=DIRECTION('',(0.121869343405148,0.,-0.992546151641322));
#9247=DIRECTION('center_axis',(0.,-1.,0.));
#9248=DIRECTION('ref_axis',(0.866025403784439,0.,-0.5));
#9249=DIRECTION('',(-0.798635510047293,0.,0.601815023152048));
#9250=DIRECTION('',(0.585429433769943,0.,0.810723367170211));
#9251=DIRECTION('',(0.551936985312059,0.,0.833885822067168));
#9252=DIRECTION('',(0.517529290979719,0.,0.855665491286186));
#9253=DIRECTION('',(0.482263407105669,0.,0.876026258834079));
#9254=DIRECTION('',(0.446197813109808,0.,0.894934361602026));
#9255=DIRECTION('',(0.40939231452609,0.,0.912358445353015));
#9256=DIRECTION('',(0.92050485345244,0.,-0.390731128489274));
#9257=DIRECTION('center_axis',(0.,-1.,0.));
#9258=DIRECTION('ref_axis',(0.866025403784439,0.,-0.5));
#9259=DIRECTION('',(-0.92050485345244,0.,-0.390731128489274));
#9260=DIRECTION('',(-0.40939231452609,0.,0.912358445353015));
#9261=DIRECTION('',(-0.446197813109808,0.,0.894934361602025));
#9262=DIRECTION('',(-0.482263407105669,0.,0.876026258834078));
#9263=DIRECTION('',(-0.51752929097972,0.,0.855665491286185));
#9264=DIRECTION('',(-0.551936985312059,0.,0.833885822067168));
#9265=DIRECTION('',(-0.585429433769943,0.,0.810723367170211));
#9266=DIRECTION('',(0.798635510047293,0.,0.601815023152048));
#9267=DIRECTION('center_axis',(0.,-1.,0.));
#9268=DIRECTION('ref_axis',(0.866025403784439,0.,-0.5));
#9269=DIRECTION('',(-0.121869343405147,0.,-0.992546151641322));
#9270=DIRECTION('',(-0.994821748296033,0.,0.101635078182804));
#9271=DIRECTION('',(-0.998134798421867,0.,0.0610485395348577));
#9272=DIRECTION('',(-0.999792698085388,0.,0.0203607675478927));
#9273=DIRECTION('',(-0.999792698085389,0.,-0.0203607675478932));
#9274=DIRECTION('',(-0.998134798421867,0.,-0.0610485395348582));
#9275=DIRECTION('',(-0.994821748296033,0.,-0.101635078182805));
#9276=DIRECTION('',(-0.121869343405148,0.,0.992546151641322));
#9277=DIRECTION('center_axis',(0.,-1.,0.));
#9278=DIRECTION('ref_axis',(0.866025403784439,0.,-0.5));
#9279=DIRECTION('',(0.798635510047293,0.,-0.601815023152048));
#9280=DIRECTION('',(-0.585429433769943,0.,-0.810723367170211));
#9281=DIRECTION('',(-0.551936985312059,0.,-0.833885822067168));
#9282=DIRECTION('',(-0.517529290979719,0.,-0.855665491286186));
#9283=DIRECTION('',(-0.482263407105669,0.,-0.876026258834078));
#9284=DIRECTION('',(-0.446197813109808,0.,-0.894934361602026));
#9285=DIRECTION('',(-0.40939231452609,0.,-0.912358445353015));
#9286=DIRECTION('',(-0.92050485345244,0.,0.390731128489274));
#9287=DIRECTION('center_axis',(0.,-1.,0.));
#9288=DIRECTION('ref_axis',(0.866025403784439,0.,-0.5));
#9289=DIRECTION('',(0.92050485345244,0.,0.390731128489275));
#9290=DIRECTION('',(0.409392314526091,0.,-0.912358445353015));
#9291=DIRECTION('',(0.446197813109809,0.,-0.894934361602025));
#9292=DIRECTION('',(0.48226340710567,0.,-0.876026258834078));
#9293=DIRECTION('',(0.51752929097972,0.,-0.855665491286185));
#9294=DIRECTION('',(0.55193698531206,0.,-0.833885822067167));
#9295=DIRECTION('',(0.585429433769943,0.,-0.81072336717021));
#9296=DIRECTION('',(-0.798635510047292,0.,-0.601815023152049));
#9297=DIRECTION('center_axis',(0.,-1.,0.));
#9298=DIRECTION('ref_axis',(0.866025403784439,0.,-0.5));
#9299=DIRECTION('center_axis',(0.,1.,0.));
#9300=DIRECTION('ref_axis',(0.866025403784439,0.,-0.5));
#9301=DIRECTION('',(0.,-1.,0.));
#9302=DIRECTION('center_axis',(0.,1.,0.));
#9303=DIRECTION('ref_axis',(0.866025403784439,0.,-0.5));
#9304=DIRECTION('',(0.,1.,0.));
#9305=DIRECTION('center_axis',(0.,1.,0.));
#9306=DIRECTION('ref_axis',(0.866025403784439,0.,-0.5));
#9307=DIRECTION('',(0.,-1.,0.));
#9308=DIRECTION('center_axis',(0.,1.,0.));
#9309=DIRECTION('ref_axis',(0.866025403784439,0.,-0.5));
#9310=DIRECTION('',(0.,1.,0.));
#9311=DIRECTION('center_axis',(0.,1.,0.));
#9312=DIRECTION('ref_axis',(0.866025403784439,0.,-0.5));
#9313=DIRECTION('',(0.,-1.,0.));
#9314=DIRECTION('center_axis',(0.,1.,0.));
#9315=DIRECTION('ref_axis',(0.866025403784439,0.,-0.5));
#9316=DIRECTION('',(0.,1.,0.));
#9317=DIRECTION('center_axis',(0.,1.,0.));
#9318=DIRECTION('ref_axis',(0.866025403784439,0.,-0.5));
#9319=DIRECTION('',(0.,1.,0.));
#9320=DIRECTION('',(0.,-1.,0.));
#9321=DIRECTION('center_axis',(0.,1.,0.));
#9322=DIRECTION('ref_axis',(0.866025403784439,0.,-0.5));
#9323=DIRECTION('center_axis',(0.,1.,0.));
#9324=DIRECTION('ref_axis',(0.866025403784439,0.,-0.5));
#9325=DIRECTION('',(0.,1.,0.));
#9326=DIRECTION('',(0.,-1.,0.));
#9327=DIRECTION('center_axis',(0.,1.,0.));
#9328=DIRECTION('ref_axis',(0.866025403784439,0.,-0.5));
#9329=DIRECTION('center_axis',(0.,1.,0.));
#9330=DIRECTION('ref_axis',(0.866025403784439,0.,-0.5));
#9331=DIRECTION('',(0.,1.,0.));
#9332=DIRECTION('',(0.,-1.,0.));
#9333=DIRECTION('center_axis',(0.,1.,0.));
#9334=DIRECTION('ref_axis',(0.866025403784439,0.,-0.5));
#9335=DIRECTION('center_axis',(0.,1.,0.));
#9336=DIRECTION('ref_axis',(0.866025403784439,0.,-0.5));
#9337=DIRECTION('',(-0.121869343405147,0.,-0.992546151641322));
#9338=DIRECTION('',(0.798635510047292,0.,0.601815023152049));
#9339=DIRECTION('',(-0.585429433769943,0.,0.81072336717021));
#9340=DIRECTION('',(-0.55193698531206,0.,0.833885822067167));
#9341=DIRECTION('',(-0.51752929097972,0.,0.855665491286185));
#9342=DIRECTION('',(-0.48226340710567,0.,0.876026258834078));
#9343=DIRECTION('',(-0.446197813109809,0.,0.894934361602025));
#9344=DIRECTION('',(-0.409392314526091,0.,0.912358445353015));
#9345=DIRECTION('',(-0.92050485345244,0.,-0.390731128489275));
#9346=DIRECTION('',(0.92050485345244,0.,-0.390731128489274));
#9347=DIRECTION('',(0.40939231452609,0.,0.912358445353015));
#9348=DIRECTION('',(0.446197813109808,0.,0.894934361602026));
#9349=DIRECTION('',(0.482263407105669,0.,0.876026258834078));
#9350=DIRECTION('',(0.517529290979719,0.,0.855665491286186));
#9351=DIRECTION('',(0.551936985312059,0.,0.833885822067168));
#9352=DIRECTION('',(0.585429433769943,0.,0.810723367170211));
#9353=DIRECTION('',(-0.798635510047293,0.,0.601815023152048));
#9354=DIRECTION('',(0.121869343405148,0.,-0.992546151641322));
#9355=DIRECTION('',(0.994821748296033,0.,0.101635078182805));
#9356=DIRECTION('',(0.998134798421867,0.,0.0610485395348582));
#9357=DIRECTION('',(0.999792698085389,0.,0.0203607675478932));
#9358=DIRECTION('',(0.999792698085388,0.,-0.0203607675478927));
#9359=DIRECTION('',(0.998134798421867,0.,-0.0610485395348577));
#9360=DIRECTION('',(0.994821748296033,0.,-0.101635078182804));
#9361=DIRECTION('',(0.121869343405147,0.,0.992546151641322));
#9362=DIRECTION('',(-0.798635510047293,0.,-0.601815023152048));
#9363=DIRECTION('',(0.585429433769943,0.,-0.810723367170211));
#9364=DIRECTION('',(0.551936985312059,0.,-0.833885822067168));
#9365=DIRECTION('',(0.51752929097972,0.,-0.855665491286185));
#9366=DIRECTION('',(0.482263407105669,0.,-0.876026258834078));
#9367=DIRECTION('',(0.446197813109808,0.,-0.894934361602025));
#9368=DIRECTION('',(0.40939231452609,0.,-0.912358445353015));
#9369=DIRECTION('',(0.92050485345244,0.,0.390731128489274));
#9370=DIRECTION('',(-0.92050485345244,0.,0.390731128489274));
#9371=DIRECTION('',(-0.40939231452609,0.,-0.912358445353015));
#9372=DIRECTION('',(-0.446197813109808,0.,-0.894934361602026));
#9373=DIRECTION('',(-0.482263407105669,0.,-0.876026258834079));
#9374=DIRECTION('',(-0.517529290979719,0.,-0.855665491286186));
#9375=DIRECTION('',(-0.551936985312059,0.,-0.833885822067168));
#9376=DIRECTION('',(-0.585429433769943,0.,-0.810723367170211));
#9377=DIRECTION('',(0.798635510047293,0.,-0.601815023152048));
#9378=DIRECTION('',(-0.121869343405148,0.,0.992546151641322));
#9379=DIRECTION('',(-0.994821748296033,0.,-0.101635078182805));
#9380=DIRECTION('',(-0.998134798421867,0.,-0.0610485395348586));
#9381=DIRECTION('',(-0.999792698085388,0.,-0.0203607675478936));
#9382=DIRECTION('',(-0.999792698085389,0.,0.0203607675478923));
#9383=DIRECTION('',(-0.998134798421867,0.,0.0610485395348574));
#9384=DIRECTION('',(-0.994821748296033,0.,0.101635078182804));
#9385=DIRECTION('center_axis',(0.390731128489275,0.,-0.92050485345244));
#9386=DIRECTION('ref_axis',(-0.92050485345244,0.,-0.390731128489275));
#9387=DIRECTION('',(0.,1.,0.));
#9388=DIRECTION('',(-0.92050485345244,0.,-0.390731128489275));
#9389=DIRECTION('',(0.,1.,0.));
#9390=DIRECTION('',(0.92050485345244,0.,0.390731128489275));
#9391=DIRECTION('',(0.,1.,0.));
#9392=DIRECTION('center_axis',(-0.912358445353015,0.,-0.409392314526091));
#9393=DIRECTION('ref_axis',(-0.409392314526091,0.,0.912358445353015));
#9394=DIRECTION('',(0.,1.,0.));
#9395=DIRECTION('',(-0.409392314526091,0.,0.912358445353015));
#9396=DIRECTION('center_axis',(-0.912358445353015,0.,-0.409392314526091));
#9397=DIRECTION('ref_axis',(-0.409392314526091,0.,0.912358445353015));
#9398=DIRECTION('',(0.409392314526091,0.,-0.912358445353015));
#9399=DIRECTION('',(0.,1.,0.));
#9400=DIRECTION('center_axis',(-0.894934361602025,0.,-0.446197813109809));
#9401=DIRECTION('ref_axis',(-0.446197813109809,0.,0.894934361602025));
#9402=DIRECTION('',(0.,1.,0.));
#9403=DIRECTION('',(-0.446197813109809,0.,0.894934361602025));
#9404=DIRECTION('center_axis',(-0.876026258834078,0.,-0.48226340710567));
#9405=DIRECTION('ref_axis',(-0.48226340710567,0.,0.876026258834078));
#9406=DIRECTION('',(0.,1.,0.));
#9407=DIRECTION('',(-0.48226340710567,0.,0.876026258834078));
#9408=DIRECTION('center_axis',(-0.855665491286185,0.,-0.51752929097972));
#9409=DIRECTION('ref_axis',(-0.51752929097972,0.,0.855665491286185));
#9410=DIRECTION('',(0.,1.,0.));
#9411=DIRECTION('',(-0.51752929097972,0.,0.855665491286185));
#9412=DIRECTION('center_axis',(-0.833885822067167,0.,-0.55193698531206));
#9413=DIRECTION('ref_axis',(-0.55193698531206,0.,0.833885822067167));
#9414=DIRECTION('',(0.,1.,0.));
#9415=DIRECTION('',(-0.55193698531206,0.,0.833885822067167));
#9416=DIRECTION('center_axis',(-0.81072336717021,0.,-0.585429433769943));
#9417=DIRECTION('ref_axis',(-0.585429433769943,0.,0.81072336717021));
#9418=DIRECTION('',(0.,-1.,0.));
#9419=DIRECTION('',(-0.585429433769944,0.,0.81072336717021));
#9420=DIRECTION('center_axis',(0.,-1.,0.));
#9421=DIRECTION('ref_axis',(0.500000000000001,0.,-0.866025403784438));
#9422=DIRECTION('',(-0.798635510047292,0.,-0.601815023152049));
#9423=DIRECTION('',(0.585429433769944,0.,-0.81072336717021));
#9424=DIRECTION('',(0.55193698531206,0.,-0.833885822067167));
#9425=DIRECTION('',(0.51752929097972,0.,-0.855665491286185));
#9426=DIRECTION('',(0.48226340710567,0.,-0.876026258834078));
#9427=DIRECTION('',(0.446197813109809,0.,-0.894934361602025));
#9428=DIRECTION('',(-0.409392314526095,0.,0.912358445353013));
#9429=DIRECTION('',(-0.446197813109808,0.,0.894934361602026));
#9430=DIRECTION('',(-0.48226340710567,0.,0.876026258834078));
#9431=DIRECTION('',(-0.51752929097972,0.,0.855665491286185));
#9432=DIRECTION('',(-0.551936985312061,0.,0.833885822067167));
#9433=DIRECTION('',(-0.58542943376994,0.,0.810723367170213));
#9434=DIRECTION('center_axis',(-0.81072336717021,0.,-0.585429433769943));
#9435=DIRECTION('ref_axis',(-0.585429433769943,0.,0.81072336717021));
#9436=DIRECTION('',(0.,1.,0.));
#9437=DIRECTION('',(0.,-1.,0.));
#9438=DIRECTION('center_axis',(-0.833885822067167,0.,-0.55193698531206));
#9439=DIRECTION('ref_axis',(-0.55193698531206,0.,0.833885822067167));
#9440=DIRECTION('',(0.,1.,0.));
#9441=DIRECTION('center_axis',(-0.855665491286185,0.,-0.51752929097972));
#9442=DIRECTION('ref_axis',(-0.51752929097972,0.,0.855665491286185));
#9443=DIRECTION('',(0.,1.,0.));
#9444=DIRECTION('center_axis',(-0.876026258834078,0.,-0.48226340710567));
#9445=DIRECTION('ref_axis',(-0.48226340710567,0.,0.876026258834078));
#9446=DIRECTION('',(0.,1.,0.));
#9447=DIRECTION('center_axis',(-0.894934361602025,0.,-0.446197813109809));
#9448=DIRECTION('ref_axis',(-0.446197813109809,0.,0.894934361602025));
#9449=DIRECTION('center_axis',(0.912358445353013,0.,0.409392314526095));
#9450=DIRECTION('ref_axis',(0.409392314526095,0.,-0.912358445353013));
#9451=DIRECTION('',(0.409392314526095,0.,-0.912358445353013));
#9452=DIRECTION('',(0.,1.,0.));
#9453=DIRECTION('center_axis',(0.894934361602026,0.,0.446197813109808));
#9454=DIRECTION('ref_axis',(0.446197813109808,0.,-0.894934361602026));
#9455=DIRECTION('',(0.446197813109808,0.,-0.894934361602026));
#9456=DIRECTION('',(0.,1.,0.));
#9457=DIRECTION('center_axis',(0.876026258834078,0.,0.48226340710567));
#9458=DIRECTION('ref_axis',(0.48226340710567,0.,-0.876026258834078));
#9459=DIRECTION('',(0.48226340710567,0.,-0.876026258834078));
#9460=DIRECTION('',(0.,1.,0.));
#9461=DIRECTION('center_axis',(0.855665491286185,0.,0.51752929097972));
#9462=DIRECTION('ref_axis',(0.51752929097972,0.,-0.855665491286185));
#9463=DIRECTION('',(0.51752929097972,0.,-0.855665491286185));
#9464=DIRECTION('',(0.,1.,0.));
#9465=DIRECTION('center_axis',(0.833885822067167,0.,0.551936985312061));
#9466=DIRECTION('ref_axis',(0.551936985312061,0.,-0.833885822067167));
#9467=DIRECTION('',(0.551936985312061,0.,-0.833885822067167));
#9468=DIRECTION('',(0.,1.,0.));
#9469=DIRECTION('center_axis',(0.810723367170213,0.,0.58542943376994));
#9470=DIRECTION('ref_axis',(0.58542943376994,0.,-0.810723367170213));
#9471=DIRECTION('',(0.58542943376994,0.,-0.810723367170213));
#9472=DIRECTION('',(0.,1.,0.));
#9473=DIRECTION('center_axis',(-0.601815023152049,0.,0.798635510047292));
#9474=DIRECTION('ref_axis',(0.798635510047292,0.,0.601815023152049));
#9475=DIRECTION('',(0.798635510047292,0.,0.601815023152049));
#9476=DIRECTION('center_axis',(0.,1.,0.));
#9477=DIRECTION('ref_axis',(-0.500000000000001,0.,0.866025403784438));
#9478=DIRECTION('center_axis',(0.601815023152048,0.,0.798635510047293));
#9479=DIRECTION('ref_axis',(0.798635510047293,0.,-0.601815023152048));
#9480=DIRECTION('',(0.,1.,0.));
#9481=DIRECTION('',(0.798635510047293,0.,-0.601815023152048));
#9482=DIRECTION('',(0.,1.,0.));
#9483=DIRECTION('',(-0.798635510047293,0.,0.601815023152048));
#9484=DIRECTION('',(0.,1.,0.));
#9485=DIRECTION('center_axis',(0.810723367170211,0.,-0.585429433769943));
#9486=DIRECTION('ref_axis',(-0.585429433769943,0.,-0.810723367170211));
#9487=DIRECTION('',(0.,1.,0.));
#9488=DIRECTION('',(-0.585429433769943,0.,-0.810723367170211));
#9489=DIRECTION('center_axis',(0.810723367170211,0.,-0.585429433769943));
#9490=DIRECTION('ref_axis',(-0.585429433769943,0.,-0.810723367170211));
#9491=DIRECTION('',(0.585429433769943,0.,0.810723367170211));
#9492=DIRECTION('',(0.,1.,0.));
#9493=DIRECTION('center_axis',(0.833885822067168,0.,-0.551936985312059));
#9494=DIRECTION('ref_axis',(-0.551936985312059,0.,-0.833885822067168));
#9495=DIRECTION('',(0.,1.,0.));
#9496=DIRECTION('',(-0.551936985312059,0.,-0.833885822067168));
#9497=DIRECTION('center_axis',(0.855665491286186,0.,-0.517529290979719));
#9498=DIRECTION('ref_axis',(-0.517529290979719,0.,-0.855665491286186));
#9499=DIRECTION('',(0.,1.,0.));
#9500=DIRECTION('',(-0.517529290979719,0.,-0.855665491286186));
#9501=DIRECTION('center_axis',(0.876026258834078,0.,-0.482263407105669));
#9502=DIRECTION('ref_axis',(-0.482263407105669,0.,-0.876026258834079));
#9503=DIRECTION('',(0.,1.,0.));
#9504=DIRECTION('',(-0.482263407105669,0.,-0.876026258834079));
#9505=DIRECTION('center_axis',(0.894934361602026,0.,-0.446197813109808));
#9506=DIRECTION('ref_axis',(-0.446197813109808,0.,-0.894934361602026));
#9507=DIRECTION('',(0.,1.,0.));
#9508=DIRECTION('',(-0.446197813109808,0.,-0.894934361602026));
#9509=DIRECTION('center_axis',(0.912358445353015,0.,-0.40939231452609));
#9510=DIRECTION('ref_axis',(-0.40939231452609,0.,-0.912358445353015));
#9511=DIRECTION('',(0.,-1.,0.));
#9512=DIRECTION('',(-0.40939231452609,0.,-0.912358445353015));
#9513=DIRECTION('center_axis',(0.,-1.,0.));
#9514=DIRECTION('ref_axis',(0.5,0.,0.866025403784439));
#9515=DIRECTION('',(0.92050485345244,0.,-0.390731128489274));
#9516=DIRECTION('',(0.40939231452609,0.,0.912358445353015));
#9517=DIRECTION('',(0.446197813109808,0.,0.894934361602026));
#9518=DIRECTION('',(0.482263407105669,0.,0.876026258834079));
#9519=DIRECTION('',(0.517529290979719,0.,0.855665491286186));
#9520=DIRECTION('',(0.551936985312059,0.,0.833885822067168));
#9521=DIRECTION('',(-0.585429433769939,0.,-0.810723367170213));
#9522=DIRECTION('',(-0.55193698531206,0.,-0.833885822067167));
#9523=DIRECTION('',(-0.517529290979719,0.,-0.855665491286186));
#9524=DIRECTION('',(-0.482263407105669,0.,-0.876026258834078));
#9525=DIRECTION('',(-0.446197813109807,0.,-0.894934361602026));
#9526=DIRECTION('',(-0.409392314526094,0.,-0.912358445353014));
#9527=DIRECTION('center_axis',(0.912358445353015,0.,-0.40939231452609));
#9528=DIRECTION('ref_axis',(-0.40939231452609,0.,-0.912358445353015));
#9529=DIRECTION('',(0.,1.,0.));
#9530=DIRECTION('',(0.,-1.,0.));
#9531=DIRECTION('center_axis',(0.894934361602026,0.,-0.446197813109808));
#9532=DIRECTION('ref_axis',(-0.446197813109808,0.,-0.894934361602026));
#9533=DIRECTION('',(0.,1.,0.));
#9534=DIRECTION('center_axis',(0.876026258834078,0.,-0.482263407105669));
#9535=DIRECTION('ref_axis',(-0.482263407105669,0.,-0.876026258834079));
#9536=DIRECTION('',(0.,1.,0.));
#9537=DIRECTION('center_axis',(0.855665491286186,0.,-0.517529290979719));
#9538=DIRECTION('ref_axis',(-0.517529290979719,0.,-0.855665491286186));
#9539=DIRECTION('',(0.,1.,0.));
#9540=DIRECTION('center_axis',(0.833885822067168,0.,-0.551936985312059));
#9541=DIRECTION('ref_axis',(-0.551936985312059,0.,-0.833885822067168));
#9542=DIRECTION('center_axis',(-0.810723367170213,0.,0.585429433769939));
#9543=DIRECTION('ref_axis',(0.585429433769939,0.,0.810723367170213));
#9544=DIRECTION('',(0.585429433769939,0.,0.810723367170213));
#9545=DIRECTION('',(0.,1.,0.));
#9546=DIRECTION('center_axis',(-0.833885822067167,0.,0.55193698531206));
#9547=DIRECTION('ref_axis',(0.55193698531206,0.,0.833885822067167));
#9548=DIRECTION('',(0.55193698531206,0.,0.833885822067167));
#9549=DIRECTION('',(0.,1.,0.));
#9550=DIRECTION('center_axis',(-0.855665491286186,0.,0.517529290979719));
#9551=DIRECTION('ref_axis',(0.517529290979719,0.,0.855665491286186));
#9552=DIRECTION('',(0.517529290979719,0.,0.855665491286186));
#9553=DIRECTION('',(0.,1.,0.));
#9554=DIRECTION('center_axis',(-0.876026258834078,0.,0.482263407105669));
#9555=DIRECTION('ref_axis',(0.482263407105669,0.,0.876026258834078));
#9556=DIRECTION('',(0.482263407105669,0.,0.876026258834078));
#9557=DIRECTION('',(0.,1.,0.));
#9558=DIRECTION('center_axis',(-0.894934361602026,0.,0.446197813109807));
#9559=DIRECTION('ref_axis',(0.446197813109807,0.,0.894934361602026));
#9560=DIRECTION('',(0.446197813109807,0.,0.894934361602026));
#9561=DIRECTION('',(0.,1.,0.));
#9562=DIRECTION('center_axis',(-0.912358445353014,0.,0.409392314526094));
#9563=DIRECTION('ref_axis',(0.409392314526094,0.,0.912358445353014));
#9564=DIRECTION('',(0.409392314526094,0.,0.912358445353014));
#9565=DIRECTION('',(0.,1.,0.));
#9566=DIRECTION('center_axis',(-0.390731128489274,0.,-0.92050485345244));
#9567=DIRECTION('ref_axis',(-0.92050485345244,0.,0.390731128489274));
#9568=DIRECTION('',(-0.92050485345244,0.,0.390731128489274));
#9569=DIRECTION('center_axis',(0.,1.,0.));
#9570=DIRECTION('ref_axis',(-0.5,0.,-0.866025403784439));
#9571=DIRECTION('center_axis',(-0.992546151641322,0.,0.121869343405147));
#9572=DIRECTION('ref_axis',(0.121869343405147,0.,0.992546151641322));
#9573=DIRECTION('',(0.,1.,0.));
#9574=DIRECTION('',(0.121869343405147,0.,0.992546151641322));
#9575=DIRECTION('',(0.,1.,0.));
#9576=DIRECTION('',(-0.121869343405147,0.,-0.992546151641322));
#9577=DIRECTION('',(0.,1.,0.));
#9578=DIRECTION('center_axis',(0.101635078182804,0.,0.994821748296033));
#9579=DIRECTION('ref_axis',(0.994821748296033,0.,-0.101635078182804));
#9580=DIRECTION('',(0.,1.,0.));
#9581=DIRECTION('',(0.994821748296033,0.,-0.101635078182804));
#9582=DIRECTION('center_axis',(0.101635078182804,0.,0.994821748296033));
#9583=DIRECTION('ref_axis',(0.994821748296033,0.,-0.101635078182804));
#9584=DIRECTION('',(-0.994821748296033,0.,0.101635078182804));
#9585=DIRECTION('',(0.,1.,0.));
#9586=DIRECTION('center_axis',(0.0610485395348577,0.,0.998134798421867));
#9587=DIRECTION('ref_axis',(0.998134798421867,0.,-0.0610485395348577));
#9588=DIRECTION('',(0.,1.,0.));
#9589=DIRECTION('',(0.998134798421867,0.,-0.0610485395348577));
#9590=DIRECTION('center_axis',(0.0203607675478927,0.,0.999792698085389));
#9591=DIRECTION('ref_axis',(0.999792698085388,0.,-0.0203607675478927));
#9592=DIRECTION('',(0.,1.,0.));
#9593=DIRECTION('',(0.999792698085388,0.,-0.0203607675478927));
#9594=DIRECTION('center_axis',(-0.0203607675478932,0.,0.999792698085389));
#9595=DIRECTION('ref_axis',(0.999792698085389,0.,0.0203607675478932));
#9596=DIRECTION('',(0.,1.,0.));
#9597=DIRECTION('',(0.999792698085389,0.,0.0203607675478932));
#9598=DIRECTION('center_axis',(-0.0610485395348582,0.,0.998134798421867));
#9599=DIRECTION('ref_axis',(0.998134798421867,0.,0.0610485395348582));
#9600=DIRECTION('',(0.,1.,0.));
#9601=DIRECTION('',(0.998134798421867,0.,0.0610485395348582));
#9602=DIRECTION('center_axis',(-0.101635078182805,0.,0.994821748296033));
#9603=DIRECTION('ref_axis',(0.994821748296033,0.,0.101635078182805));
#9604=DIRECTION('',(0.,-1.,0.));
#9605=DIRECTION('',(0.994821748296033,0.,0.101635078182805));
#9606=DIRECTION('center_axis',(0.,-1.,0.));
#9607=DIRECTION('ref_axis',(-1.,0.,-2.22044604925031E-16));
#9608=DIRECTION('',(-0.121869343405148,0.,0.992546151641322));
#9609=DIRECTION('',(-0.994821748296033,0.,-0.101635078182805));
#9610=DIRECTION('',(-0.998134798421867,0.,-0.0610485395348582));
#9611=DIRECTION('',(-0.999792698085389,0.,-0.0203607675478932));
#9612=DIRECTION('',(-0.999792698085388,0.,0.0203607675478927));
#9613=DIRECTION('',(-0.998134798421867,0.,0.0610485395348577));
#9614=DIRECTION('',(0.994821748296033,0.,-0.1016350781828));
#9615=DIRECTION('',(0.998134798421867,0.,-0.0610485395348589));
#9616=DIRECTION('',(0.999792698085388,0.,-0.0203607675478925));
#9617=DIRECTION('',(0.999792698085389,0.,0.0203607675478929));
#9618=DIRECTION('',(0.998134798421867,0.,0.0610485395348593));
#9619=DIRECTION('',(0.994821748296033,0.,0.1016350781828));
#9620=DIRECTION('center_axis',(-0.101635078182805,0.,0.994821748296033));
#9621=DIRECTION('ref_axis',(0.994821748296033,0.,0.101635078182805));
#9622=DIRECTION('',(0.,1.,0.));
#9623=DIRECTION('',(0.,-1.,0.));
#9624=DIRECTION('center_axis',(-0.0610485395348582,0.,0.998134798421867));
#9625=DIRECTION('ref_axis',(0.998134798421867,0.,0.0610485395348582));
#9626=DIRECTION('',(0.,1.,0.));
#9627=DIRECTION('center_axis',(-0.0203607675478932,0.,0.999792698085389));
#9628=DIRECTION('ref_axis',(0.999792698085389,0.,0.0203607675478932));
#9629=DIRECTION('',(0.,1.,0.));
#9630=DIRECTION('center_axis',(0.0203607675478927,0.,0.999792698085389));
#9631=DIRECTION('ref_axis',(0.999792698085388,0.,-0.0203607675478927));
#9632=DIRECTION('',(0.,1.,0.));
#9633=DIRECTION('center_axis',(0.0610485395348577,0.,0.998134798421867));
#9634=DIRECTION('ref_axis',(0.998134798421867,0.,-0.0610485395348577));
#9635=DIRECTION('center_axis',(-0.1016350781828,0.,-0.994821748296033));
#9636=DIRECTION('ref_axis',(-0.994821748296033,0.,0.1016350781828));
#9637=DIRECTION('',(-0.994821748296033,0.,0.1016350781828));
#9638=DIRECTION('',(0.,1.,0.));
#9639=DIRECTION('center_axis',(-0.0610485395348589,0.,-0.998134798421867));
#9640=DIRECTION('ref_axis',(-0.998134798421867,0.,0.0610485395348589));
#9641=DIRECTION('',(-0.998134798421867,0.,0.0610485395348589));
#9642=DIRECTION('',(0.,1.,0.));
#9643=DIRECTION('center_axis',(-0.0203607675478925,0.,-0.999792698085389));
#9644=DIRECTION('ref_axis',(-0.999792698085388,0.,0.0203607675478925));
#9645=DIRECTION('',(-0.999792698085388,0.,0.0203607675478925));
#9646=DIRECTION('',(0.,1.,0.));
#9647=DIRECTION('center_axis',(0.0203607675478929,0.,-0.999792698085389));
#9648=DIRECTION('ref_axis',(-0.999792698085389,0.,-0.0203607675478929));
#9649=DIRECTION('',(-0.999792698085389,0.,-0.0203607675478929));
#9650=DIRECTION('',(0.,1.,0.));
#9651=DIRECTION('center_axis',(0.0610485395348593,0.,-0.998134798421867));
#9652=DIRECTION('ref_axis',(-0.998134798421867,0.,-0.0610485395348593));
#9653=DIRECTION('',(-0.998134798421867,0.,-0.0610485395348593));
#9654=DIRECTION('',(0.,1.,0.));
#9655=DIRECTION('center_axis',(0.1016350781828,0.,-0.994821748296033));
#9656=DIRECTION('ref_axis',(-0.994821748296033,0.,-0.1016350781828));
#9657=DIRECTION('',(-0.994821748296033,0.,-0.1016350781828));
#9658=DIRECTION('',(0.,1.,0.));
#9659=DIRECTION('center_axis',(0.992546151641322,0.,0.121869343405148));
#9660=DIRECTION('ref_axis',(0.121869343405148,0.,-0.992546151641322));
#9661=DIRECTION('',(0.121869343405148,0.,-0.992546151641322));
#9662=DIRECTION('center_axis',(0.,1.,0.));
#9663=DIRECTION('ref_axis',(1.,0.,2.22044604925031E-16));
#9664=DIRECTION('center_axis',(-0.601815023152048,0.,-0.798635510047293));
#9665=DIRECTION('ref_axis',(-0.798635510047293,0.,0.601815023152048));
#9666=DIRECTION('',(0.,1.,0.));
#9667=DIRECTION('',(-0.798635510047293,0.,0.601815023152048));
#9668=DIRECTION('',(0.,1.,0.));
#9669=DIRECTION('',(0.798635510047293,0.,-0.601815023152048));
#9670=DIRECTION('',(0.,1.,0.));
#9671=DIRECTION('center_axis',(-0.810723367170211,0.,0.585429433769943));
#9672=DIRECTION('ref_axis',(0.585429433769943,0.,0.810723367170211));
#9673=DIRECTION('',(0.,1.,0.));
#9674=DIRECTION('',(0.585429433769943,0.,0.810723367170211));
#9675=DIRECTION('center_axis',(-0.810723367170211,0.,0.585429433769943));
#9676=DIRECTION('ref_axis',(0.585429433769943,0.,0.810723367170211));
#9677=DIRECTION('',(-0.585429433769943,0.,-0.810723367170211));
#9678=DIRECTION('',(0.,1.,0.));
#9679=DIRECTION('center_axis',(-0.833885822067168,0.,0.551936985312059));
#9680=DIRECTION('ref_axis',(0.551936985312059,0.,0.833885822067168));
#9681=DIRECTION('',(0.,1.,0.));
#9682=DIRECTION('',(0.551936985312059,0.,0.833885822067168));
#9683=DIRECTION('center_axis',(-0.855665491286186,0.,0.517529290979719));
#9684=DIRECTION('ref_axis',(0.517529290979719,0.,0.855665491286186));
#9685=DIRECTION('',(0.,1.,0.));
#9686=DIRECTION('',(0.517529290979719,0.,0.855665491286186));
#9687=DIRECTION('center_axis',(-0.876026258834078,0.,0.482263407105669));
#9688=DIRECTION('ref_axis',(0.482263407105669,0.,0.876026258834078));
#9689=DIRECTION('',(0.,1.,0.));
#9690=DIRECTION('',(0.482263407105669,0.,0.876026258834078));
#9691=DIRECTION('center_axis',(-0.894934361602026,0.,0.446197813109808));
#9692=DIRECTION('ref_axis',(0.446197813109808,0.,0.894934361602026));
#9693=DIRECTION('',(0.,1.,0.));
#9694=DIRECTION('',(0.446197813109808,0.,0.894934361602026));
#9695=DIRECTION('center_axis',(-0.912358445353015,0.,0.40939231452609));
#9696=DIRECTION('ref_axis',(0.40939231452609,0.,0.912358445353015));
#9697=DIRECTION('',(0.,-1.,0.));
#9698=DIRECTION('',(0.40939231452609,0.,0.912358445353015));
#9699=DIRECTION('center_axis',(0.,-1.,0.));
#9700=DIRECTION('ref_axis',(-0.5,0.,-0.866025403784439));
#9701=DIRECTION('',(-0.92050485345244,0.,0.390731128489274));
#9702=DIRECTION('',(-0.40939231452609,0.,-0.912358445353015));
#9703=DIRECTION('',(-0.446197813109808,0.,-0.894934361602026));
#9704=DIRECTION('',(-0.482263407105669,0.,-0.876026258834078));
#9705=DIRECTION('',(-0.517529290979719,0.,-0.855665491286186));
#9706=DIRECTION('',(-0.551936985312059,0.,-0.833885822067168));
#9707=DIRECTION('',(0.585429433769939,0.,0.810723367170213));
#9708=DIRECTION('',(0.55193698531206,0.,0.833885822067167));
#9709=DIRECTION('',(0.517529290979719,0.,0.855665491286186));
#9710=DIRECTION('',(0.482263407105669,0.,0.876026258834078));
#9711=DIRECTION('',(0.446197813109807,0.,0.894934361602026));
#9712=DIRECTION('',(0.409392314526094,0.,0.912358445353014));
#9713=DIRECTION('center_axis',(-0.912358445353015,0.,0.40939231452609));
#9714=DIRECTION('ref_axis',(0.40939231452609,0.,0.912358445353015));
#9715=DIRECTION('',(0.,1.,0.));
#9716=DIRECTION('',(0.,-1.,0.));
#9717=DIRECTION('center_axis',(-0.894934361602026,0.,0.446197813109808));
#9718=DIRECTION('ref_axis',(0.446197813109808,0.,0.894934361602026));
#9719=DIRECTION('',(0.,1.,0.));
#9720=DIRECTION('center_axis',(-0.876026258834078,0.,0.482263407105669));
#9721=DIRECTION('ref_axis',(0.482263407105669,0.,0.876026258834078));
#9722=DIRECTION('',(0.,1.,0.));
#9723=DIRECTION('center_axis',(-0.855665491286186,0.,0.517529290979719));
#9724=DIRECTION('ref_axis',(0.517529290979719,0.,0.855665491286186));
#9725=DIRECTION('',(0.,1.,0.));
#9726=DIRECTION('center_axis',(-0.833885822067168,0.,0.551936985312059));
#9727=DIRECTION('ref_axis',(0.551936985312059,0.,0.833885822067168));
#9728=DIRECTION('center_axis',(0.810723367170213,0.,-0.585429433769939));
#9729=DIRECTION('ref_axis',(-0.585429433769939,0.,-0.810723367170213));
#9730=DIRECTION('',(-0.585429433769939,0.,-0.810723367170213));
#9731=DIRECTION('',(0.,1.,0.));
#9732=DIRECTION('center_axis',(0.833885822067167,0.,-0.55193698531206));
#9733=DIRECTION('ref_axis',(-0.55193698531206,0.,-0.833885822067167));
#9734=DIRECTION('',(-0.55193698531206,0.,-0.833885822067167));
#9735=DIRECTION('',(0.,1.,0.));
#9736=DIRECTION('center_axis',(0.855665491286186,0.,-0.517529290979719));
#9737=DIRECTION('ref_axis',(-0.517529290979719,0.,-0.855665491286186));
#9738=DIRECTION('',(-0.517529290979719,0.,-0.855665491286186));
#9739=DIRECTION('',(0.,1.,0.));
#9740=DIRECTION('center_axis',(0.876026258834078,0.,-0.482263407105669));
#9741=DIRECTION('ref_axis',(-0.482263407105669,0.,-0.876026258834078));
#9742=DIRECTION('',(-0.482263407105669,0.,-0.876026258834078));
#9743=DIRECTION('',(0.,1.,0.));
#9744=DIRECTION('center_axis',(0.894934361602026,0.,-0.446197813109807));
#9745=DIRECTION('ref_axis',(-0.446197813109807,0.,-0.894934361602026));
#9746=DIRECTION('',(-0.446197813109807,0.,-0.894934361602026));
#9747=DIRECTION('',(0.,1.,0.));
#9748=DIRECTION('center_axis',(0.912358445353014,0.,-0.409392314526094));
#9749=DIRECTION('ref_axis',(-0.409392314526094,0.,-0.912358445353014));
#9750=DIRECTION('',(-0.409392314526094,0.,-0.912358445353014));
#9751=DIRECTION('',(0.,1.,0.));
#9752=DIRECTION('center_axis',(0.390731128489274,0.,0.92050485345244));
#9753=DIRECTION('ref_axis',(0.92050485345244,0.,-0.390731128489274));
#9754=DIRECTION('',(0.92050485345244,0.,-0.390731128489274));
#9755=DIRECTION('center_axis',(0.,1.,0.));
#9756=DIRECTION('ref_axis',(0.5,0.,0.866025403784439));
#9757=DIRECTION('center_axis',(-0.390731128489274,0.,0.92050485345244));
#9758=DIRECTION('ref_axis',(0.92050485345244,0.,0.390731128489274));
#9759=DIRECTION('',(0.,1.,0.));
#9760=DIRECTION('',(0.92050485345244,0.,0.390731128489274));
#9761=DIRECTION('',(0.,1.,0.));
#9762=DIRECTION('',(-0.92050485345244,0.,-0.390731128489274));
#9763=DIRECTION('',(0.,1.,0.));
#9764=DIRECTION('center_axis',(0.912358445353015,0.,0.40939231452609));
#9765=DIRECTION('ref_axis',(0.40939231452609,0.,-0.912358445353015));
#9766=DIRECTION('',(0.,1.,0.));
#9767=DIRECTION('',(0.40939231452609,0.,-0.912358445353015));
#9768=DIRECTION('center_axis',(0.912358445353015,0.,0.40939231452609));
#9769=DIRECTION('ref_axis',(0.40939231452609,0.,-0.912358445353015));
#9770=DIRECTION('',(-0.40939231452609,0.,0.912358445353015));
#9771=DIRECTION('',(0.,1.,0.));
#9772=DIRECTION('center_axis',(0.894934361602025,0.,0.446197813109808));
#9773=DIRECTION('ref_axis',(0.446197813109808,0.,-0.894934361602025));
#9774=DIRECTION('',(0.,1.,0.));
#9775=DIRECTION('',(0.446197813109808,0.,-0.894934361602025));
#9776=DIRECTION('center_axis',(0.876026258834078,0.,0.482263407105669));
#9777=DIRECTION('ref_axis',(0.482263407105669,0.,-0.876026258834078));
#9778=DIRECTION('',(0.,1.,0.));
#9779=DIRECTION('',(0.482263407105669,0.,-0.876026258834078));
#9780=DIRECTION('center_axis',(0.855665491286185,0.,0.51752929097972));
#9781=DIRECTION('ref_axis',(0.51752929097972,0.,-0.855665491286185));
#9782=DIRECTION('',(0.,1.,0.));
#9783=DIRECTION('',(0.51752929097972,0.,-0.855665491286185));
#9784=DIRECTION('center_axis',(0.833885822067168,0.,0.551936985312059));
#9785=DIRECTION('ref_axis',(0.551936985312059,0.,-0.833885822067168));
#9786=DIRECTION('',(0.,1.,0.));
#9787=DIRECTION('',(0.551936985312059,0.,-0.833885822067167));
#9788=DIRECTION('center_axis',(0.810723367170211,0.,0.585429433769943));
#9789=DIRECTION('ref_axis',(0.585429433769943,0.,-0.810723367170211));
#9790=DIRECTION('',(0.,-1.,0.));
#9791=DIRECTION('',(0.585429433769943,0.,-0.810723367170211));
#9792=DIRECTION('center_axis',(0.,-1.,0.));
#9793=DIRECTION('ref_axis',(-0.5,0.,0.866025403784439));
#9794=DIRECTION('',(0.798635510047293,0.,0.601815023152048));
#9795=DIRECTION('',(-0.585429433769943,0.,0.810723367170211));
#9796=DIRECTION('',(-0.551936985312059,0.,0.833885822067167));
#9797=DIRECTION('',(-0.51752929097972,0.,0.855665491286185));
#9798=DIRECTION('',(-0.482263407105669,0.,0.876026258834078));
#9799=DIRECTION('',(-0.446197813109808,0.,0.894934361602025));
#9800=DIRECTION('',(0.409392314526094,0.,-0.912358445353013));
#9801=DIRECTION('',(0.446197813109807,0.,-0.894934361602026));
#9802=DIRECTION('',(0.48226340710567,0.,-0.876026258834078));
#9803=DIRECTION('',(0.517529290979719,0.,-0.855665491286185));
#9804=DIRECTION('',(0.55193698531206,0.,-0.833885822067167));
#9805=DIRECTION('',(0.58542943376994,0.,-0.810723367170213));
#9806=DIRECTION('center_axis',(0.810723367170211,0.,0.585429433769943));
#9807=DIRECTION('ref_axis',(0.585429433769943,0.,-0.810723367170211));
#9808=DIRECTION('',(0.,1.,0.));
#9809=DIRECTION('',(0.,-1.,0.));
#9810=DIRECTION('center_axis',(0.833885822067168,0.,0.551936985312059));
#9811=DIRECTION('ref_axis',(0.551936985312059,0.,-0.833885822067168));
#9812=DIRECTION('',(0.,1.,0.));
#9813=DIRECTION('center_axis',(0.855665491286185,0.,0.51752929097972));
#9814=DIRECTION('ref_axis',(0.51752929097972,0.,-0.855665491286185));
#9815=DIRECTION('',(0.,1.,0.));
#9816=DIRECTION('center_axis',(0.876026258834078,0.,0.482263407105669));
#9817=DIRECTION('ref_axis',(0.482263407105669,0.,-0.876026258834078));
#9818=DIRECTION('',(0.,1.,0.));
#9819=DIRECTION('center_axis',(0.894934361602025,0.,0.446197813109808));
#9820=DIRECTION('ref_axis',(0.446197813109808,0.,-0.894934361602025));
#9821=DIRECTION('center_axis',(-0.912358445353013,0.,-0.409392314526094));
#9822=DIRECTION('ref_axis',(-0.409392314526094,0.,0.912358445353013));
#9823=DIRECTION('',(-0.409392314526094,0.,0.912358445353013));
#9824=DIRECTION('',(0.,1.,0.));
#9825=DIRECTION('center_axis',(-0.894934361602026,0.,-0.446197813109807));
#9826=DIRECTION('ref_axis',(-0.446197813109807,0.,0.894934361602026));
#9827=DIRECTION('',(-0.446197813109807,0.,0.894934361602026));
#9828=DIRECTION('',(0.,1.,0.));
#9829=DIRECTION('center_axis',(-0.876026258834078,0.,-0.48226340710567));
#9830=DIRECTION('ref_axis',(-0.48226340710567,0.,0.876026258834078));
#9831=DIRECTION('',(-0.48226340710567,0.,0.876026258834078));
#9832=DIRECTION('',(0.,1.,0.));
#9833=DIRECTION('center_axis',(-0.855665491286185,0.,-0.517529290979719));
#9834=DIRECTION('ref_axis',(-0.517529290979719,0.,0.855665491286185));
#9835=DIRECTION('',(-0.517529290979719,0.,0.855665491286185));
#9836=DIRECTION('',(0.,1.,0.));
#9837=DIRECTION('center_axis',(-0.833885822067167,0.,-0.55193698531206));
#9838=DIRECTION('ref_axis',(-0.55193698531206,0.,0.833885822067167));
#9839=DIRECTION('',(-0.55193698531206,0.,0.833885822067167));
#9840=DIRECTION('',(0.,1.,0.));
#9841=DIRECTION('center_axis',(-0.810723367170213,0.,-0.585429433769939));
#9842=DIRECTION('ref_axis',(-0.585429433769939,0.,0.810723367170213));
#9843=DIRECTION('',(-0.58542943376994,0.,0.810723367170213));
#9844=DIRECTION('',(0.,1.,0.));
#9845=DIRECTION('center_axis',(0.601815023152048,0.,-0.798635510047293));
#9846=DIRECTION('ref_axis',(-0.798635510047293,0.,-0.601815023152048));
#9847=DIRECTION('',(-0.798635510047293,0.,-0.601815023152048));
#9848=DIRECTION('center_axis',(0.,1.,0.));
#9849=DIRECTION('ref_axis',(0.5,0.,-0.866025403784439));
#9850=DIRECTION('center_axis',(0.992546151641322,0.,-0.121869343405147));
#9851=DIRECTION('ref_axis',(-0.121869343405147,0.,-0.992546151641322));
#9852=DIRECTION('',(0.,1.,0.));
#9853=DIRECTION('',(-0.121869343405147,0.,-0.992546151641322));
#9854=DIRECTION('',(0.,1.,0.));
#9855=DIRECTION('',(0.121869343405147,0.,0.992546151641322));
#9856=DIRECTION('',(0.,1.,0.));
#9857=DIRECTION('center_axis',(-0.101635078182804,0.,-0.994821748296033));
#9858=DIRECTION('ref_axis',(-0.994821748296033,0.,0.101635078182804));
#9859=DIRECTION('',(0.,1.,0.));
#9860=DIRECTION('',(-0.994821748296033,0.,0.101635078182804));
#9861=DIRECTION('center_axis',(-0.101635078182804,0.,-0.994821748296033));
#9862=DIRECTION('ref_axis',(-0.994821748296033,0.,0.101635078182804));
#9863=DIRECTION('',(0.994821748296033,0.,-0.101635078182804));
#9864=DIRECTION('',(0.,1.,0.));
#9865=DIRECTION('center_axis',(-0.0610485395348574,0.,-0.998134798421867));
#9866=DIRECTION('ref_axis',(-0.998134798421867,0.,0.0610485395348574));
#9867=DIRECTION('',(0.,1.,0.));
#9868=DIRECTION('',(-0.998134798421867,0.,0.0610485395348574));
#9869=DIRECTION('center_axis',(-0.0203607675478923,0.,-0.999792698085389));
#9870=DIRECTION('ref_axis',(-0.999792698085389,0.,0.0203607675478923));
#9871=DIRECTION('',(0.,1.,0.));
#9872=DIRECTION('',(-0.999792698085389,0.,0.0203607675478923));
#9873=DIRECTION('center_axis',(0.0203607675478936,0.,-0.999792698085388));
#9874=DIRECTION('ref_axis',(-0.999792698085388,0.,-0.0203607675478936));
#9875=DIRECTION('',(0.,1.,0.));
#9876=DIRECTION('',(-0.999792698085388,0.,-0.0203607675478936));
#9877=DIRECTION('center_axis',(0.0610485395348586,0.,-0.998134798421867));
#9878=DIRECTION('ref_axis',(-0.998134798421867,0.,-0.0610485395348586));
#9879=DIRECTION('',(0.,1.,0.));
#9880=DIRECTION('',(-0.998134798421867,0.,-0.0610485395348586));
#9881=DIRECTION('center_axis',(0.101635078182805,0.,-0.994821748296033));
#9882=DIRECTION('ref_axis',(-0.994821748296033,0.,-0.101635078182805));
#9883=DIRECTION('',(0.,-1.,0.));
#9884=DIRECTION('',(-0.994821748296033,0.,-0.101635078182805));
#9885=DIRECTION('center_axis',(0.,-1.,0.));
#9886=DIRECTION('ref_axis',(1.,0.,6.10622663543836E-16));
#9887=DIRECTION('',(0.121869343405148,0.,-0.992546151641322));
#9888=DIRECTION('',(0.994821748296033,0.,0.101635078182805));
#9889=DIRECTION('',(0.998134798421867,0.,0.0610485395348586));
#9890=DIRECTION('',(0.999792698085388,0.,0.0203607675478936));
#9891=DIRECTION('',(0.999792698085389,0.,-0.0203607675478923));
#9892=DIRECTION('',(0.998134798421867,0.,-0.0610485395348574));
#9893=DIRECTION('',(-0.994821748296033,0.,0.1016350781828));
#9894=DIRECTION('',(-0.998134798421867,0.,0.0610485395348585));
#9895=DIRECTION('',(-0.999792698085389,0.,0.0203607675478921));
#9896=DIRECTION('',(-0.999792698085388,0.,-0.0203607675478933));
#9897=DIRECTION('',(-0.998134798421867,0.,-0.0610485395348597));
#9898=DIRECTION('',(-0.994821748296033,0.,-0.101635078182801));
#9899=DIRECTION('center_axis',(0.101635078182805,0.,-0.994821748296033));
#9900=DIRECTION('ref_axis',(-0.994821748296033,0.,-0.101635078182805));
#9901=DIRECTION('',(0.,1.,0.));
#9902=DIRECTION('',(0.,-1.,0.));
#9903=DIRECTION('center_axis',(0.0610485395348586,0.,-0.998134798421867));
#9904=DIRECTION('ref_axis',(-0.998134798421867,0.,-0.0610485395348586));
#9905=DIRECTION('',(0.,1.,0.));
#9906=DIRECTION('center_axis',(0.0203607675478936,0.,-0.999792698085388));
#9907=DIRECTION('ref_axis',(-0.999792698085388,0.,-0.0203607675478936));
#9908=DIRECTION('',(0.,1.,0.));
#9909=DIRECTION('center_axis',(-0.0203607675478923,0.,-0.999792698085389));
#9910=DIRECTION('ref_axis',(-0.999792698085389,0.,0.0203607675478923));
#9911=DIRECTION('',(0.,1.,0.));
#9912=DIRECTION('center_axis',(-0.0610485395348574,0.,-0.998134798421867));
#9913=DIRECTION('ref_axis',(-0.998134798421867,0.,0.0610485395348574));
#9914=DIRECTION('center_axis',(0.1016350781828,0.,0.994821748296033));
#9915=DIRECTION('ref_axis',(0.994821748296033,0.,-0.1016350781828));
#9916=DIRECTION('',(0.994821748296033,0.,-0.1016350781828));
#9917=DIRECTION('',(0.,1.,0.));
#9918=DIRECTION('center_axis',(0.0610485395348585,0.,0.998134798421867));
#9919=DIRECTION('ref_axis',(0.998134798421867,0.,-0.0610485395348585));
#9920=DIRECTION('',(0.998134798421867,0.,-0.0610485395348585));
#9921=DIRECTION('',(0.,1.,0.));
#9922=DIRECTION('center_axis',(0.0203607675478921,0.,0.999792698085389));
#9923=DIRECTION('ref_axis',(0.999792698085389,0.,-0.0203607675478921));
#9924=DIRECTION('',(0.999792698085389,0.,-0.0203607675478921));
#9925=DIRECTION('',(0.,1.,0.));
#9926=DIRECTION('center_axis',(-0.0203607675478933,0.,0.999792698085389));
#9927=DIRECTION('ref_axis',(0.999792698085388,0.,0.0203607675478933));
#9928=DIRECTION('',(0.999792698085388,0.,0.0203607675478933));
#9929=DIRECTION('',(0.,1.,0.));
#9930=DIRECTION('center_axis',(-0.0610485395348597,0.,0.998134798421867));
#9931=DIRECTION('ref_axis',(0.998134798421867,0.,0.0610485395348597));
#9932=DIRECTION('',(0.998134798421867,0.,0.0610485395348597));
#9933=DIRECTION('',(0.,1.,0.));
#9934=DIRECTION('center_axis',(-0.101635078182801,0.,0.994821748296033));
#9935=DIRECTION('ref_axis',(0.994821748296033,0.,0.101635078182801));
#9936=DIRECTION('',(0.994821748296033,0.,0.101635078182801));
#9937=DIRECTION('',(0.,1.,0.));
#9938=DIRECTION('center_axis',(-0.992546151641322,0.,-0.121869343405148));
#9939=DIRECTION('ref_axis',(-0.121869343405148,0.,0.992546151641322));
#9940=DIRECTION('',(-0.121869343405148,0.,0.992546151641322));
#9941=DIRECTION('center_axis',(0.,1.,0.));
#9942=DIRECTION('ref_axis',(-1.,0.,-6.10622663543836E-16));
#11410=CARTESIAN_POINT('',(0.,0.,0.));
#11411=CARTESIAN_POINT('Origin',(0.,-0.4,0.));
#11412=CARTESIAN_POINT('',(0.0994453842185998,-0.4,0.809917659739319));
#11413=CARTESIAN_POINT('',(0.099567253562005,-0.4,0.81091020589096));
#11414=CARTESIAN_POINT('',(0.0818108902278751,-0.4,0.666296231596819));
#11415=CARTESIAN_POINT('',(0.0663886785289718,-0.4,0.813294868644317));
#11416=CARTESIAN_POINT('',(0.091181207796194,-0.4,0.810761961965568));
#11417=CARTESIAN_POINT('',(0.0332218842499737,-0.4,0.815323436684413));
#11418=CARTESIAN_POINT('',(0.0580969799592227,-0.4,0.813802010654341));
#11419=CARTESIAN_POINT('',(-4.9960036108132E-16,-0.4,0.816));
#11420=CARTESIAN_POINT('',(0.0249164131874799,-0.4,0.81549257751331));
#11421=CARTESIAN_POINT('',(-0.0332218842499747,-0.4,0.815323436684413));
#11422=CARTESIAN_POINT('',(-0.00830547106249374,-0.4,0.815830859171103));
#11423=CARTESIAN_POINT('',(-0.0663886785289729,-0.4,0.813294868644317));
#11424=CARTESIAN_POINT('',(-0.0415135828197248,-0.4,0.814816294674389));
#11425=CARTESIAN_POINT('',(-0.0994453842186008,-0.4,0.809917659739319));
#11426=CARTESIAN_POINT('',(-0.074652854951381,-0.4,0.812450566418067));
#11427=CARTESIAN_POINT('',(-0.099567253562006,-0.4,0.81091020589096));
#11428=CARTESIAN_POINT('',(-0.0497226921093004,-0.4,0.404958829869659));
#11429=CARTESIAN_POINT('',(-0.652485211708638,-0.4,0.491682873915223));
#11430=CARTESIAN_POINT('Origin',(0.,-0.4,0.));
#11431=CARTESIAN_POINT('',(-0.651686576198591,-0.4,0.491081058892071));
#11432=CARTESIAN_POINT('',(-0.536124017894748,-0.4,0.40399842504197));
#11433=CARTESIAN_POINT('',(-0.671139677749021,-0.4,0.464141716451927));
#11434=CARTESIAN_POINT('',(-0.656549851586198,-0.4,0.484346223282036));
#11435=CARTESIAN_POINT('',(-0.689479866344548,-0.4,0.43643271406427));
#11436=CARTESIAN_POINT('',(-0.675724724897902,-0.4,0.457214465855013));
#11437=CARTESIAN_POINT('',(-0.706676729488102,-0.4,0.408));
#11438=CARTESIAN_POINT('',(-0.693779082130436,-0.4,0.429324535548202));
#11439=CARTESIAN_POINT('',(-0.722701750594522,-0.4,0.378890722620142));
#11440=CARTESIAN_POINT('',(-0.710682984764707,-0.4,0.400722680655036));
#11441=CARTESIAN_POINT('',(-0.737528356277993,-0.4,0.34915315219239));
#11442=CARTESIAN_POINT('',(-0.72640840201539,-0.4,0.371456330013204));
#11443=CARTESIAN_POINT('',(-0.751131960417191,-0.4,0.318836600847247));
#11444=CARTESIAN_POINT('',(-0.740929257312793,-0.4,0.341574014356103));
#11445=CARTESIAN_POINT('',(-0.752052465270644,-0.4,0.319227331975736));
#11446=CARTESIAN_POINT('',(-0.375565980208596,-0.4,0.159418300423624));
#11447=CARTESIAN_POINT('',(-0.752052465270644,-0.4,-0.319227331975737));
#11448=CARTESIAN_POINT('Origin',(0.,-0.4,0.));
#11449=CARTESIAN_POINT('',(-0.751131960417191,-0.4,-0.318836600847248));
#11450=CARTESIAN_POINT('',(-0.617934908122623,-0.4,-0.26229780655485));
#11451=CARTESIAN_POINT('',(-0.737528356277993,-0.4,-0.34915315219239));
#11452=CARTESIAN_POINT('',(-0.747731059382392,-0.4,-0.326415738683532));
#11453=CARTESIAN_POINT('',(-0.722701750594522,-0.4,-0.378890722620143));
#11454=CARTESIAN_POINT('',(-0.733821704857125,-0.4,-0.356587544799328));
#11455=CARTESIAN_POINT('',(-0.706676729488102,-0.4,-0.408));
#11456=CARTESIAN_POINT('',(-0.718695495317917,-0.4,-0.386168041965107));
#11457=CARTESIAN_POINT('',(-0.689479866344548,-0.4,-0.43643271406427));
#11458=CARTESIAN_POINT('',(-0.702377513702213,-0.4,-0.415108178516068));
#11459=CARTESIAN_POINT('',(-0.67113967774902,-0.4,-0.464141716451927));
#11460=CARTESIAN_POINT('',(-0.684894819195665,-0.4,-0.443359964661185));
#11461=CARTESIAN_POINT('',(-0.651686576198591,-0.4,-0.491081058892072));
#11462=CARTESIAN_POINT('',(-0.666276402361412,-0.4,-0.470876552061964));
#11463=CARTESIAN_POINT('',(-0.652485211708638,-0.4,-0.491682873915224));
#11464=CARTESIAN_POINT('',(-0.325843288099295,-0.4,-0.245540529446036));
#11465=CARTESIAN_POINT('',(-0.0995672535620054,-0.4,-0.81091020589096));
#11466=CARTESIAN_POINT('Origin',(0.,-0.4,0.));
#11467=CARTESIAN_POINT('',(-0.0994453842186002,-0.4,-0.809917659739319));
#11468=CARTESIAN_POINT('',(-0.0818108902278754,-0.4,-0.666296231596819));
#11469=CARTESIAN_POINT('',(-0.0663886785289722,-0.4,-0.813294868644317));
#11470=CARTESIAN_POINT('',(-0.0911812077961943,-0.4,-0.810761961965568));
#11471=CARTESIAN_POINT('',(-0.033221884249974,-0.4,-0.815323436684413));
#11472=CARTESIAN_POINT('',(-0.0580969799592231,-0.4,-0.813802010654341));
#11473=CARTESIAN_POINT('',(2.22044604925031E-16,-0.4,-0.816));
#11474=CARTESIAN_POINT('',(-0.0249164131874803,-0.4,-0.81549257751331));
#11475=CARTESIAN_POINT('',(0.0332218842499744,-0.4,-0.815323436684413));
#11476=CARTESIAN_POINT('',(0.00830547106249352,-0.4,-0.815830859171103));
#11477=CARTESIAN_POINT('',(0.0663886785289726,-0.4,-0.813294868644317));
#11478=CARTESIAN_POINT('',(0.0415135828197244,-0.4,-0.814816294674389));
#11479=CARTESIAN_POINT('',(0.0994453842186005,-0.4,-0.809917659739319));
#11480=CARTESIAN_POINT('',(0.0746528549513807,-0.4,-0.812450566418067));
#11481=CARTESIAN_POINT('',(0.0995672535620056,-0.4,-0.81091020589096));
#11482=CARTESIAN_POINT('',(0.0497226921093002,-0.4,-0.404958829869659));
#11483=CARTESIAN_POINT('',(0.652485211708638,-0.4,-0.491682873915223));
#11484=CARTESIAN_POINT('Origin',(0.,-0.4,0.));
#11485=CARTESIAN_POINT('',(0.651686576198591,-0.4,-0.491081058892071));
#11486=CARTESIAN_POINT('',(0.536124017894748,-0.4,-0.40399842504197));
#11487=CARTESIAN_POINT('',(0.67113967774902,-0.4,-0.464141716451927));
#11488=CARTESIAN_POINT('',(0.656549851586198,-0.4,-0.484346223282036));
#11489=CARTESIAN_POINT('',(0.689479866344548,-0.4,-0.43643271406427));
#11490=CARTESIAN_POINT('',(0.675724724897902,-0.4,-0.457214465855013));
#11491=CARTESIAN_POINT('',(0.706676729488102,-0.4,-0.408));
#11492=CARTESIAN_POINT('',(0.693779082130436,-0.4,-0.429324535548202));
#11493=CARTESIAN_POINT('',(0.722701750594522,-0.4,-0.378890722620142));
#11494=CARTESIAN_POINT('',(0.710682984764707,-0.4,-0.400722680655036));
#11495=CARTESIAN_POINT('',(0.737528356277993,-0.4,-0.34915315219239));
#11496=CARTESIAN_POINT('',(0.72640840201539,-0.4,-0.371456330013204));
#11497=CARTESIAN_POINT('',(0.751131960417191,-0.4,-0.318836600847247));
#11498=CARTESIAN_POINT('',(0.740929257312793,-0.4,-0.341574014356103));
#11499=CARTESIAN_POINT('',(0.752052465270644,-0.4,-0.319227331975737));
#11500=CARTESIAN_POINT('',(0.375565980208596,-0.4,-0.159418300423624));
#11501=CARTESIAN_POINT('',(0.752052465270643,-0.4,0.319227331975737));
#11502=CARTESIAN_POINT('Origin',(0.,-0.4,0.));
#11503=CARTESIAN_POINT('',(0.751131960417191,-0.4,0.318836600847248));
#11504=CARTESIAN_POINT('',(0.617934908122623,-0.4,0.26229780655485));
#11505=CARTESIAN_POINT('',(0.737528356277993,-0.4,0.349153152192391));
#11506=CARTESIAN_POINT('',(0.747731059382392,-0.4,0.326415738683533));
#11507=CARTESIAN_POINT('',(0.722701750594521,-0.4,0.378890722620143));
#11508=CARTESIAN_POINT('',(0.733821704857125,-0.4,0.356587544799328));
#11509=CARTESIAN_POINT('',(0.706676729488102,-0.4,0.408000000000001));
#11510=CARTESIAN_POINT('',(0.718695495317916,-0.4,0.386168041965108));
#11511=CARTESIAN_POINT('',(0.689479866344547,-0.4,0.436432714064271));
#11512=CARTESIAN_POINT('',(0.702377513702213,-0.4,0.415108178516068));
#11513=CARTESIAN_POINT('',(0.67113967774902,-0.4,0.464141716451928));
#11514=CARTESIAN_POINT('',(0.684894819195665,-0.4,0.443359964661185));
#11515=CARTESIAN_POINT('',(0.65168657619859,-0.4,0.491081058892072));
#11516=CARTESIAN_POINT('',(0.666276402361412,-0.4,0.470876552061965));
#11517=CARTESIAN_POINT('',(0.652485211708638,-0.4,0.491682873915224));
#11518=CARTESIAN_POINT('',(0.325843288099295,-0.4,0.245540529446036));
#11519=CARTESIAN_POINT('Origin',(0.,-0.4,0.));
#11520=CARTESIAN_POINT('Origin',(0.,0.,0.));
#11521=CARTESIAN_POINT('',(0.752052465270644,0.4,-0.319227331975737));
#11522=CARTESIAN_POINT('',(0.752052465270644,0.,-0.319227331975737));
#11523=CARTESIAN_POINT('',(0.752052465270643,0.4,0.319227331975737));
#11524=CARTESIAN_POINT('Origin',(0.,0.4,0.));
#11525=CARTESIAN_POINT('',(0.752052465270643,0.,0.319227331975737));
#11526=CARTESIAN_POINT('Origin',(0.,0.,0.));
#11527=CARTESIAN_POINT('',(-0.099567253562006,0.4,0.81091020589096));
#11528=CARTESIAN_POINT('',(-0.099567253562006,0.,0.81091020589096));
#11529=CARTESIAN_POINT('',(-0.652485211708638,0.4,0.491682873915223));
#11530=CARTESIAN_POINT('Origin',(0.,0.4,0.));
#11531=CARTESIAN_POINT('',(-0.652485211708638,0.,0.491682873915223));
#11532=CARTESIAN_POINT('Origin',(0.,0.,0.));
#11533=CARTESIAN_POINT('',(-0.652485211708638,0.4,-0.491682873915224));
#11534=CARTESIAN_POINT('',(-0.652485211708638,0.,-0.491682873915224));
#11535=CARTESIAN_POINT('',(-0.0995672535620054,0.4,-0.81091020589096));
#11536=CARTESIAN_POINT('Origin',(0.,0.4,0.));
#11537=CARTESIAN_POINT('',(-0.0995672535620054,0.,-0.81091020589096));
#11538=CARTESIAN_POINT('Origin',(0.,0.,0.));
#11539=CARTESIAN_POINT('',(0.652485211708638,0.4,-0.491682873915223));
#11540=CARTESIAN_POINT('',(0.652485211708638,0.,-0.491682873915223));
#11541=CARTESIAN_POINT('',(0.0995672535620056,0.4,-0.81091020589096));
#11542=CARTESIAN_POINT('',(0.0995672535620056,0.,-0.81091020589096));
#11543=CARTESIAN_POINT('Origin',(0.,0.4,0.));
#11544=CARTESIAN_POINT('Origin',(0.,0.,0.));
#11545=CARTESIAN_POINT('',(-0.752052465270644,0.4,-0.319227331975737));
#11546=CARTESIAN_POINT('',(-0.752052465270644,0.,-0.319227331975737));
#11547=CARTESIAN_POINT('',(-0.752052465270644,0.4,0.319227331975736));
#11548=CARTESIAN_POINT('',(-0.752052465270644,0.,0.319227331975736));
#11549=CARTESIAN_POINT('Origin',(0.,0.4,0.));
#11550=CARTESIAN_POINT('Origin',(0.,0.,0.));
#11551=CARTESIAN_POINT('',(0.099567253562005,0.4,0.81091020589096));
#11552=CARTESIAN_POINT('',(0.099567253562005,0.,0.81091020589096));
#11553=CARTESIAN_POINT('',(0.652485211708638,0.4,0.491682873915224));
#11554=CARTESIAN_POINT('',(0.652485211708638,0.,0.491682873915224));
#11555=CARTESIAN_POINT('Origin',(0.,0.4,0.));
#11556=CARTESIAN_POINT('Origin',(0.,0.4,0.));
#11557=CARTESIAN_POINT('',(0.0994453842185998,0.4,0.809917659739319));
#11558=CARTESIAN_POINT('',(0.0818108902278751,0.4,0.666296231596819));
#11559=CARTESIAN_POINT('',(0.65168657619859,0.4,0.491081058892072));
#11560=CARTESIAN_POINT('',(0.325843288099295,0.4,0.245540529446036));
#11561=CARTESIAN_POINT('',(0.67113967774902,0.4,0.464141716451928));
#11562=CARTESIAN_POINT('',(0.666276402361412,0.4,0.470876552061965));
#11563=CARTESIAN_POINT('',(0.689479866344547,0.4,0.436432714064271));
#11564=CARTESIAN_POINT('',(0.684894819195665,0.4,0.443359964661185));
#11565=CARTESIAN_POINT('',(0.706676729488102,0.4,0.408000000000001));
#11566=CARTESIAN_POINT('',(0.702377513702213,0.4,0.415108178516068));
#11567=CARTESIAN_POINT('',(0.722701750594521,0.4,0.378890722620143));
#11568=CARTESIAN_POINT('',(0.718695495317916,0.4,0.386168041965108));
#11569=CARTESIAN_POINT('',(0.737528356277993,0.4,0.349153152192391));
#11570=CARTESIAN_POINT('',(0.733821704857125,0.4,0.356587544799328));
#11571=CARTESIAN_POINT('',(0.751131960417191,0.4,0.318836600847248));
#11572=CARTESIAN_POINT('',(0.747731059382392,0.4,0.326415738683533));
#11573=CARTESIAN_POINT('',(0.617934908122623,0.4,0.26229780655485));
#11574=CARTESIAN_POINT('',(0.751131960417191,0.4,-0.318836600847247));
#11575=CARTESIAN_POINT('',(0.375565980208596,0.4,-0.159418300423624));
#11576=CARTESIAN_POINT('',(0.737528356277993,0.4,-0.34915315219239));
#11577=CARTESIAN_POINT('',(0.740929257312793,0.4,-0.341574014356103));
#11578=CARTESIAN_POINT('',(0.722701750594522,0.4,-0.378890722620142));
#11579=CARTESIAN_POINT('',(0.72640840201539,0.4,-0.371456330013204));
#11580=CARTESIAN_POINT('',(0.706676729488102,0.4,-0.408));
#11581=CARTESIAN_POINT('',(0.710682984764707,0.4,-0.400722680655036));
#11582=CARTESIAN_POINT('',(0.689479866344548,0.4,-0.43643271406427));
#11583=CARTESIAN_POINT('',(0.693779082130436,0.4,-0.429324535548202));
#11584=CARTESIAN_POINT('',(0.67113967774902,0.4,-0.464141716451927));
#11585=CARTESIAN_POINT('',(0.675724724897902,0.4,-0.457214465855013));
#11586=CARTESIAN_POINT('',(0.651686576198591,0.4,-0.491081058892071));
#11587=CARTESIAN_POINT('',(0.656549851586198,0.4,-0.484346223282036));
#11588=CARTESIAN_POINT('',(0.536124017894748,0.4,-0.40399842504197));
#11589=CARTESIAN_POINT('',(0.0994453842186005,0.4,-0.809917659739319));
#11590=CARTESIAN_POINT('',(0.0497226921093002,0.4,-0.404958829869659));
#11591=CARTESIAN_POINT('',(0.0663886785289726,0.4,-0.813294868644317));
#11592=CARTESIAN_POINT('',(0.0746528549513807,0.4,-0.812450566418067));
#11593=CARTESIAN_POINT('',(0.0332218842499744,0.4,-0.815323436684413));
#11594=CARTESIAN_POINT('',(0.0415135828197244,0.4,-0.814816294674389));
#11595=CARTESIAN_POINT('',(2.22044604925031E-16,0.4,-0.816));
#11596=CARTESIAN_POINT('',(0.00830547106249352,0.4,-0.815830859171103));
#11597=CARTESIAN_POINT('',(-0.033221884249974,0.4,-0.815323436684413));
#11598=CARTESIAN_POINT('',(-0.0249164131874803,0.4,-0.81549257751331));
#11599=CARTESIAN_POINT('',(-0.0663886785289722,0.4,-0.813294868644317));
#11600=CARTESIAN_POINT('',(-0.0580969799592231,0.4,-0.813802010654341));
#11601=CARTESIAN_POINT('',(-0.0994453842186002,0.4,-0.809917659739319));
#11602=CARTESIAN_POINT('',(-0.0911812077961943,0.4,-0.810761961965568));
#11603=CARTESIAN_POINT('',(-0.0818108902278754,0.4,-0.666296231596819));
#11604=CARTESIAN_POINT('',(-0.651686576198591,0.4,-0.491081058892072));
#11605=CARTESIAN_POINT('',(-0.325843288099295,0.4,-0.245540529446036));
#11606=CARTESIAN_POINT('',(-0.67113967774902,0.4,-0.464141716451927));
#11607=CARTESIAN_POINT('',(-0.666276402361412,0.4,-0.470876552061964));
#11608=CARTESIAN_POINT('',(-0.689479866344548,0.4,-0.43643271406427));
#11609=CARTESIAN_POINT('',(-0.684894819195665,0.4,-0.443359964661185));
#11610=CARTESIAN_POINT('',(-0.706676729488102,0.4,-0.408));
#11611=CARTESIAN_POINT('',(-0.702377513702213,0.4,-0.415108178516068));
#11612=CARTESIAN_POINT('',(-0.722701750594522,0.4,-0.378890722620143));
#11613=CARTESIAN_POINT('',(-0.718695495317917,0.4,-0.386168041965107));
#11614=CARTESIAN_POINT('',(-0.737528356277993,0.4,-0.34915315219239));
#11615=CARTESIAN_POINT('',(-0.733821704857125,0.4,-0.356587544799328));
#11616=CARTESIAN_POINT('',(-0.751131960417191,0.4,-0.318836600847248));
#11617=CARTESIAN_POINT('',(-0.747731059382392,0.4,-0.326415738683532));
#11618=CARTESIAN_POINT('',(-0.617934908122623,0.4,-0.26229780655485));
#11619=CARTESIAN_POINT('',(-0.751131960417191,0.4,0.318836600847247));
#11620=CARTESIAN_POINT('',(-0.375565980208596,0.4,0.159418300423624));
#11621=CARTESIAN_POINT('',(-0.737528356277993,0.4,0.34915315219239));
#11622=CARTESIAN_POINT('',(-0.740929257312793,0.4,0.341574014356103));
#11623=CARTESIAN_POINT('',(-0.722701750594522,0.4,0.378890722620142));
#11624=CARTESIAN_POINT('',(-0.72640840201539,0.4,0.371456330013204));
#11625=CARTESIAN_POINT('',(-0.706676729488102,0.4,0.408));
#11626=CARTESIAN_POINT('',(-0.710682984764707,0.4,0.400722680655036));
#11627=CARTESIAN_POINT('',(-0.689479866344548,0.4,0.43643271406427));
#11628=CARTESIAN_POINT('',(-0.693779082130436,0.4,0.429324535548202));
#11629=CARTESIAN_POINT('',(-0.671139677749021,0.4,0.464141716451927));
#11630=CARTESIAN_POINT('',(-0.675724724897902,0.4,0.457214465855013));
#11631=CARTESIAN_POINT('',(-0.651686576198591,0.4,0.491081058892071));
#11632=CARTESIAN_POINT('',(-0.656549851586198,0.4,0.484346223282036));
#11633=CARTESIAN_POINT('',(-0.536124017894748,0.4,0.40399842504197));
#11634=CARTESIAN_POINT('',(-0.0994453842186008,0.4,0.809917659739319));
#11635=CARTESIAN_POINT('',(-0.0497226921093004,0.4,0.404958829869659));
#11636=CARTESIAN_POINT('',(-0.0663886785289729,0.4,0.813294868644317));
#11637=CARTESIAN_POINT('',(-0.074652854951381,0.4,0.812450566418067));
#11638=CARTESIAN_POINT('',(-0.0332218842499747,0.4,0.815323436684413));
#11639=CARTESIAN_POINT('',(-0.0415135828197248,0.4,0.814816294674389));
#11640=CARTESIAN_POINT('',(-4.9960036108132E-16,0.4,0.816));
#11641=CARTESIAN_POINT('',(-0.00830547106249374,0.4,0.815830859171103));
#11642=CARTESIAN_POINT('',(0.0332218842499737,0.4,0.815323436684413));
#11643=CARTESIAN_POINT('',(0.0249164131874799,0.4,0.81549257751331));
#11644=CARTESIAN_POINT('',(0.0663886785289718,0.4,0.813294868644317));
#11645=CARTESIAN_POINT('',(0.0580969799592227,0.4,0.813802010654341));
#11646=CARTESIAN_POINT('',(0.091181207796194,0.4,0.810761961965568));
#11647=CARTESIAN_POINT('Origin',(1.23586981624525,0.,0.5245956131097));
#11648=CARTESIAN_POINT('',(0.751131960417191,1.,0.318836600847248));
#11649=CARTESIAN_POINT('',(0.751131960417191,0.,0.318836600847248));
#11650=CARTESIAN_POINT('',(1.23586981624525,1.,0.5245956131097));
#11651=CARTESIAN_POINT('',(1.23586981624525,1.,0.5245956131097));
#11652=CARTESIAN_POINT('',(1.23586981624525,-1.,0.5245956131097));
#11653=CARTESIAN_POINT('',(1.23586981624525,0.,0.5245956131097));
#11654=CARTESIAN_POINT('',(0.751131960417191,-1.,0.318836600847248));
#11655=CARTESIAN_POINT('',(1.23586981624525,-1.,0.5245956131097));
#11656=CARTESIAN_POINT('',(0.751131960417191,0.,0.318836600847248));
#11657=CARTESIAN_POINT('Origin',(0.751131960417191,0.,0.318836600847248));
#11658=CARTESIAN_POINT('',(0.737528356277993,1.,0.349153152192391));
#11659=CARTESIAN_POINT('',(0.737528356277993,0.,0.349153152192391));
#11660=CARTESIAN_POINT('',(0.751131960417191,1.,0.318836600847248));
#11661=CARTESIAN_POINT('Origin',(0.751131960417191,0.,0.318836600847248));
#11662=CARTESIAN_POINT('',(0.737528356277993,-1.,0.349153152192391));
#11663=CARTESIAN_POINT('',(0.751131960417191,-1.,0.318836600847248));
#11664=CARTESIAN_POINT('',(0.737528356277993,0.,0.349153152192391));
#11665=CARTESIAN_POINT('Origin',(0.737528356277993,0.,0.349153152192391));
#11666=CARTESIAN_POINT('',(0.722701750594521,1.,0.378890722620143));
#11667=CARTESIAN_POINT('',(0.722701750594521,0.,0.378890722620143));
#11668=CARTESIAN_POINT('',(0.737528356277993,1.,0.349153152192391));
#11669=CARTESIAN_POINT('Origin',(0.722701750594521,0.,0.378890722620143));
#11670=CARTESIAN_POINT('',(0.706676729488102,1.,0.408000000000001));
#11671=CARTESIAN_POINT('',(0.706676729488102,0.,0.408000000000001));
#11672=CARTESIAN_POINT('',(0.722701750594521,1.,0.378890722620143));
#11673=CARTESIAN_POINT('Origin',(0.706676729488102,0.,0.408000000000001));
#11674=CARTESIAN_POINT('',(0.689479866344547,1.,0.436432714064271));
#11675=CARTESIAN_POINT('',(0.689479866344547,0.,0.436432714064271));
#11676=CARTESIAN_POINT('',(0.706676729488102,1.,0.408000000000001));
#11677=CARTESIAN_POINT('Origin',(0.689479866344547,0.,0.436432714064271));
#11678=CARTESIAN_POINT('',(0.67113967774902,1.,0.464141716451928));
#11679=CARTESIAN_POINT('',(0.67113967774902,0.,0.464141716451928));
#11680=CARTESIAN_POINT('',(0.689479866344547,1.,0.436432714064271));
#11681=CARTESIAN_POINT('Origin',(0.67113967774902,0.,0.464141716451928));
#11682=CARTESIAN_POINT('',(0.65168657619859,1.,0.491081058892072));
#11683=CARTESIAN_POINT('',(0.65168657619859,0.,0.491081058892072));
#11684=CARTESIAN_POINT('',(0.67113967774902,1.,0.464141716451928));
#11685=CARTESIAN_POINT('Origin',(0.932067487714439,-1.,0.53812941493483));
#11686=CARTESIAN_POINT('',(1.07224803578949,-1.,0.807996850083941));
#11687=CARTESIAN_POINT('',(0.65168657619859,-1.,0.491081058892072));
#11688=CARTESIAN_POINT('',(0.65168657619859,-1.,0.491081058892072));
#11689=CARTESIAN_POINT('',(0.67113967774902,-1.,0.464141716451928));
#11690=CARTESIAN_POINT('',(0.67113967774902,-1.,0.464141716451928));
#11691=CARTESIAN_POINT('',(0.689479866344547,-1.,0.436432714064271));
#11692=CARTESIAN_POINT('',(0.689479866344547,-1.,0.436432714064271));
#11693=CARTESIAN_POINT('',(0.706676729488102,-1.,0.408000000000001));
#11694=CARTESIAN_POINT('',(0.706676729488102,-1.,0.408000000000001));
#11695=CARTESIAN_POINT('',(0.722701750594521,-1.,0.378890722620143));
#11696=CARTESIAN_POINT('',(0.722701750594521,-1.,0.378890722620143));
#11697=CARTESIAN_POINT('',(0.737528356277993,-1.,0.349153152192391));
#11698=CARTESIAN_POINT('',(1.21348721953288,-1.,0.574476742810666));
#11699=CARTESIAN_POINT('',(1.21348721953288,-1.,0.574476742810666));
#11700=CARTESIAN_POINT('',(1.1890923656228,-1.,0.623405250232603));
#11701=CARTESIAN_POINT('',(1.1890923656228,-1.,0.623405250232603));
#11702=CARTESIAN_POINT('',(1.16272570712099,-1.,0.671300000000001));
#11703=CARTESIAN_POINT('',(1.16272570712099,-1.,0.671300000000001));
#11704=CARTESIAN_POINT('',(1.13443096636543,-1.,0.718081570959179));
#11705=CARTESIAN_POINT('',(1.13443096636543,-1.,0.718081570959179));
#11706=CARTESIAN_POINT('',(1.10425506292382,-1.,0.76367238787789));
#11707=CARTESIAN_POINT('',(1.10425506292382,-1.,0.76367238787789));
#11708=CARTESIAN_POINT('',(1.07224803578949,-1.,0.807996850083941));
#11709=CARTESIAN_POINT('Origin',(0.67113967774902,0.,0.464141716451928));
#11710=CARTESIAN_POINT('',(0.67113967774902,0.,0.464141716451928));
#11711=CARTESIAN_POINT('',(0.65168657619859,0.,0.491081058892072));
#11712=CARTESIAN_POINT('Origin',(0.689479866344547,0.,0.436432714064271));
#11713=CARTESIAN_POINT('',(0.689479866344547,0.,0.436432714064271));
#11714=CARTESIAN_POINT('Origin',(0.706676729488102,0.,0.408000000000001));
#11715=CARTESIAN_POINT('',(0.706676729488102,0.,0.408000000000001));
#11716=CARTESIAN_POINT('Origin',(0.722701750594521,0.,0.378890722620143));
#11717=CARTESIAN_POINT('',(0.722701750594521,0.,0.378890722620143));
#11718=CARTESIAN_POINT('Origin',(0.737528356277993,0.,0.349153152192391));
#11719=CARTESIAN_POINT('Origin',(1.21348721953288,0.,0.574476742810666));
#11720=CARTESIAN_POINT('',(1.21348721953288,1.,0.574476742810666));
#11721=CARTESIAN_POINT('',(1.21348721953288,1.,0.574476742810666));
#11722=CARTESIAN_POINT('',(1.21348721953288,0.,0.574476742810666));
#11723=CARTESIAN_POINT('Origin',(1.1890923656228,0.,0.623405250232603));
#11724=CARTESIAN_POINT('',(1.1890923656228,1.,0.623405250232603));
#11725=CARTESIAN_POINT('',(1.1890923656228,1.,0.623405250232603));
#11726=CARTESIAN_POINT('',(1.1890923656228,0.,0.623405250232603));
#11727=CARTESIAN_POINT('Origin',(1.16272570712099,0.,0.671300000000001));
#11728=CARTESIAN_POINT('',(1.16272570712099,1.,0.671300000000001));
#11729=CARTESIAN_POINT('',(1.16272570712099,1.,0.671300000000001));
#11730=CARTESIAN_POINT('',(1.16272570712099,0.,0.671300000000001));
#11731=CARTESIAN_POINT('Origin',(1.13443096636543,0.,0.718081570959179));
#11732=CARTESIAN_POINT('',(1.13443096636543,1.,0.718081570959179));
#11733=CARTESIAN_POINT('',(1.13443096636543,1.,0.718081570959179));
#11734=CARTESIAN_POINT('',(1.13443096636543,0.,0.718081570959179));
#11735=CARTESIAN_POINT('Origin',(1.10425506292382,0.,0.76367238787789));
#11736=CARTESIAN_POINT('',(1.10425506292382,1.,0.76367238787789));
#11737=CARTESIAN_POINT('',(1.10425506292382,1.,0.76367238787789));
#11738=CARTESIAN_POINT('',(1.10425506292382,0.,0.76367238787789));
#11739=CARTESIAN_POINT('Origin',(1.07224803578949,0.,0.807996850083941));
#11740=CARTESIAN_POINT('',(1.07224803578949,1.,0.807996850083941));
#11741=CARTESIAN_POINT('',(1.07224803578949,1.,0.807996850083941));
#11742=CARTESIAN_POINT('',(1.07224803578949,0.,0.807996850083941));
#11743=CARTESIAN_POINT('Origin',(0.65168657619859,0.,0.491081058892072));
#11744=CARTESIAN_POINT('',(0.65168657619859,1.,0.491081058892072));
#11745=CARTESIAN_POINT('Origin',(0.932067487714439,1.,0.53812941493483));
#11746=CARTESIAN_POINT('Origin',(-1.0722480357895,0.,0.80799685008394));
#11747=CARTESIAN_POINT('',(-0.651686576198591,1.,0.491081058892071));
#11748=CARTESIAN_POINT('',(-0.651686576198591,0.,0.491081058892071));
#11749=CARTESIAN_POINT('',(-1.0722480357895,1.,0.80799685008394));
#11750=CARTESIAN_POINT('',(-1.0722480357895,1.,0.80799685008394));
#11751=CARTESIAN_POINT('',(-1.0722480357895,-1.,0.80799685008394));
#11752=CARTESIAN_POINT('',(-1.0722480357895,0.,0.80799685008394));
#11753=CARTESIAN_POINT('',(-0.651686576198591,-1.,0.491081058892071));
#11754=CARTESIAN_POINT('',(-1.0722480357895,-1.,0.80799685008394));
#11755=CARTESIAN_POINT('',(-0.651686576198591,0.,0.491081058892071));
#11756=CARTESIAN_POINT('Origin',(-0.651686576198591,0.,0.491081058892071));
#11757=CARTESIAN_POINT('',(-0.671139677749021,1.,0.464141716451927));
#11758=CARTESIAN_POINT('',(-0.671139677749021,0.,0.464141716451927));
#11759=CARTESIAN_POINT('',(-0.651686576198591,1.,0.491081058892071));
#11760=CARTESIAN_POINT('Origin',(-0.651686576198591,0.,0.491081058892071));
#11761=CARTESIAN_POINT('',(-0.671139677749021,-1.,0.464141716451927));
#11762=CARTESIAN_POINT('',(-0.651686576198591,-1.,0.491081058892071));
#11763=CARTESIAN_POINT('',(-0.671139677749021,0.,0.464141716451927));
#11764=CARTESIAN_POINT('Origin',(-0.671139677749021,0.,0.464141716451927));
#11765=CARTESIAN_POINT('',(-0.689479866344548,1.,0.43643271406427));
#11766=CARTESIAN_POINT('',(-0.689479866344548,0.,0.43643271406427));
#11767=CARTESIAN_POINT('',(-0.671139677749021,1.,0.464141716451927));
#11768=CARTESIAN_POINT('Origin',(-0.689479866344548,0.,0.43643271406427));
#11769=CARTESIAN_POINT('',(-0.706676729488102,1.,0.408));
#11770=CARTESIAN_POINT('',(-0.706676729488102,0.,0.408));
#11771=CARTESIAN_POINT('',(-0.689479866344548,1.,0.43643271406427));
#11772=CARTESIAN_POINT('Origin',(-0.706676729488102,0.,0.408));
#11773=CARTESIAN_POINT('',(-0.722701750594522,1.,0.378890722620142));
#11774=CARTESIAN_POINT('',(-0.722701750594522,0.,0.378890722620142));
#11775=CARTESIAN_POINT('',(-0.706676729488102,1.,0.408));
#11776=CARTESIAN_POINT('Origin',(-0.722701750594522,0.,0.378890722620142));
#11777=CARTESIAN_POINT('',(-0.737528356277993,1.,0.34915315219239));
#11778=CARTESIAN_POINT('',(-0.737528356277993,0.,0.34915315219239));
#11779=CARTESIAN_POINT('',(-0.722701750594522,1.,0.378890722620142));
#11780=CARTESIAN_POINT('Origin',(-0.737528356277993,0.,0.34915315219239));
#11781=CARTESIAN_POINT('',(-0.751131960417191,1.,0.318836600847247));
#11782=CARTESIAN_POINT('',(-0.751131960417191,0.,0.318836600847247));
#11783=CARTESIAN_POINT('',(-0.737528356277993,1.,0.34915315219239));
#11784=CARTESIAN_POINT('Origin',(-0.932067487714439,-1.,0.538129414934829));
#11785=CARTESIAN_POINT('',(-1.23586981624525,-1.,0.524595613109699));
#11786=CARTESIAN_POINT('',(-0.751131960417191,-1.,0.318836600847247));
#11787=CARTESIAN_POINT('',(-0.751131960417191,-1.,0.318836600847247));
#11788=CARTESIAN_POINT('',(-0.737528356277993,-1.,0.34915315219239));
#11789=CARTESIAN_POINT('',(-0.737528356277993,-1.,0.34915315219239));
#11790=CARTESIAN_POINT('',(-0.722701750594522,-1.,0.378890722620142));
#11791=CARTESIAN_POINT('',(-0.722701750594522,-1.,0.378890722620142));
#11792=CARTESIAN_POINT('',(-0.706676729488102,-1.,0.408));
#11793=CARTESIAN_POINT('',(-0.706676729488102,-1.,0.408));
#11794=CARTESIAN_POINT('',(-0.689479866344548,-1.,0.43643271406427));
#11795=CARTESIAN_POINT('',(-0.689479866344548,-1.,0.43643271406427));
#11796=CARTESIAN_POINT('',(-0.671139677749021,-1.,0.464141716451927));
#11797=CARTESIAN_POINT('',(-1.10425506292382,-1.,0.763672387877888));
#11798=CARTESIAN_POINT('',(-1.10425506292382,-1.,0.763672387877888));
#11799=CARTESIAN_POINT('',(-1.13443096636543,-1.,0.718081570959177));
#11800=CARTESIAN_POINT('',(-1.13443096636543,-1.,0.718081570959177));
#11801=CARTESIAN_POINT('',(-1.16272570712099,-1.,0.6713));
#11802=CARTESIAN_POINT('',(-1.16272570712099,-1.,0.6713));
#11803=CARTESIAN_POINT('',(-1.1890923656228,-1.,0.623405250232602));
#11804=CARTESIAN_POINT('',(-1.1890923656228,-1.,0.623405250232602));
#11805=CARTESIAN_POINT('',(-1.21348721953288,-1.,0.574476742810665));
#11806=CARTESIAN_POINT('',(-1.21348721953288,-1.,0.574476742810665));
#11807=CARTESIAN_POINT('',(-1.23586981624525,-1.,0.524595613109699));
#11808=CARTESIAN_POINT('Origin',(-0.737528356277993,0.,0.34915315219239));
#11809=CARTESIAN_POINT('',(-0.737528356277993,0.,0.34915315219239));
#11810=CARTESIAN_POINT('',(-0.751131960417191,0.,0.318836600847247));
#11811=CARTESIAN_POINT('Origin',(-0.722701750594522,0.,0.378890722620142));
#11812=CARTESIAN_POINT('',(-0.722701750594522,0.,0.378890722620142));
#11813=CARTESIAN_POINT('Origin',(-0.706676729488102,0.,0.408));
#11814=CARTESIAN_POINT('',(-0.706676729488102,0.,0.408));
#11815=CARTESIAN_POINT('Origin',(-0.689479866344548,0.,0.43643271406427));
#11816=CARTESIAN_POINT('',(-0.689479866344548,0.,0.43643271406427));
#11817=CARTESIAN_POINT('Origin',(-0.671139677749021,0.,0.464141716451927));
#11818=CARTESIAN_POINT('Origin',(-1.10425506292382,0.,0.763672387877888));
#11819=CARTESIAN_POINT('',(-1.10425506292382,1.,0.763672387877888));
#11820=CARTESIAN_POINT('',(-1.10425506292382,1.,0.763672387877888));
#11821=CARTESIAN_POINT('',(-1.10425506292382,0.,0.763672387877888));
#11822=CARTESIAN_POINT('Origin',(-1.13443096636543,0.,0.718081570959177));
#11823=CARTESIAN_POINT('',(-1.13443096636543,1.,0.718081570959177));
#11824=CARTESIAN_POINT('',(-1.13443096636543,1.,0.718081570959177));
#11825=CARTESIAN_POINT('',(-1.13443096636543,0.,0.718081570959177));
#11826=CARTESIAN_POINT('Origin',(-1.16272570712099,0.,0.6713));
#11827=CARTESIAN_POINT('',(-1.16272570712099,1.,0.6713));
#11828=CARTESIAN_POINT('',(-1.16272570712099,1.,0.6713));
#11829=CARTESIAN_POINT('',(-1.16272570712099,0.,0.6713));
#11830=CARTESIAN_POINT('Origin',(-1.1890923656228,0.,0.623405250232602));
#11831=CARTESIAN_POINT('',(-1.1890923656228,1.,0.623405250232602));
#11832=CARTESIAN_POINT('',(-1.1890923656228,1.,0.623405250232602));
#11833=CARTESIAN_POINT('',(-1.1890923656228,0.,0.623405250232602));
#11834=CARTESIAN_POINT('Origin',(-1.21348721953288,0.,0.574476742810665));
#11835=CARTESIAN_POINT('',(-1.21348721953288,1.,0.574476742810665));
#11836=CARTESIAN_POINT('',(-1.21348721953288,1.,0.574476742810665));
#11837=CARTESIAN_POINT('',(-1.21348721953288,0.,0.574476742810665));
#11838=CARTESIAN_POINT('Origin',(-1.23586981624525,0.,0.524595613109699));
#11839=CARTESIAN_POINT('',(-1.23586981624525,1.,0.524595613109699));
#11840=CARTESIAN_POINT('',(-1.23586981624525,1.,0.524595613109699));
#11841=CARTESIAN_POINT('',(-1.23586981624525,0.,0.524595613109699));
#11842=CARTESIAN_POINT('Origin',(-0.751131960417191,0.,0.318836600847247));
#11843=CARTESIAN_POINT('',(-0.751131960417191,1.,0.318836600847247));
#11844=CARTESIAN_POINT('Origin',(-0.932067487714439,1.,0.538129414934829));
#11845=CARTESIAN_POINT('Origin',(-0.163621780455751,0.,-1.33259246319364));
#11846=CARTESIAN_POINT('',(-0.0994453842186002,1.,-0.809917659739319));
#11847=CARTESIAN_POINT('',(-0.0994453842186002,0.,-0.809917659739319));
#11848=CARTESIAN_POINT('',(-0.163621780455751,1.,-1.33259246319364));
#11849=CARTESIAN_POINT('',(-0.163621780455751,1.,-1.33259246319364));
#11850=CARTESIAN_POINT('',(-0.163621780455751,-1.,-1.33259246319364));
#11851=CARTESIAN_POINT('',(-0.163621780455751,0.,-1.33259246319364));
#11852=CARTESIAN_POINT('',(-0.0994453842186002,-1.,-0.809917659739319));
#11853=CARTESIAN_POINT('',(-0.163621780455751,-1.,-1.33259246319364));
#11854=CARTESIAN_POINT('',(-0.0994453842186002,0.,-0.809917659739319));
#11855=CARTESIAN_POINT('Origin',(-0.0994453842186002,0.,-0.809917659739319));
#11856=CARTESIAN_POINT('',(-0.0663886785289722,1.,-0.813294868644317));
#11857=CARTESIAN_POINT('',(-0.0663886785289722,0.,-0.813294868644317));
#11858=CARTESIAN_POINT('',(-0.0994453842186002,1.,-0.809917659739319));
#11859=CARTESIAN_POINT('Origin',(-0.0994453842186002,0.,-0.809917659739319));
#11860=CARTESIAN_POINT('',(-0.0663886785289722,-1.,-0.813294868644317));
#11861=CARTESIAN_POINT('',(-0.0994453842186002,-1.,-0.809917659739319));
#11862=CARTESIAN_POINT('',(-0.0663886785289722,0.,-0.813294868644317));
#11863=CARTESIAN_POINT('Origin',(-0.0663886785289722,0.,-0.813294868644317));
#11864=CARTESIAN_POINT('',(-0.033221884249974,1.,-0.815323436684413));
#11865=CARTESIAN_POINT('',(-0.033221884249974,0.,-0.815323436684413));
#11866=CARTESIAN_POINT('',(-0.0663886785289722,1.,-0.813294868644317));
#11867=CARTESIAN_POINT('Origin',(-0.033221884249974,0.,-0.815323436684413));
#11868=CARTESIAN_POINT('',(2.22044604925031E-16,1.,-0.816));
#11869=CARTESIAN_POINT('',(2.22044604925031E-16,0.,-0.816));
#11870=CARTESIAN_POINT('',(-0.033221884249974,1.,-0.815323436684413));
#11871=CARTESIAN_POINT('Origin',(2.22044604925031E-16,0.,-0.816));
#11872=CARTESIAN_POINT('',(0.0332218842499744,1.,-0.815323436684413));
#11873=CARTESIAN_POINT('',(0.0332218842499744,0.,-0.815323436684413));
#11874=CARTESIAN_POINT('',(2.22044604925031E-16,1.,-0.816));
#11875=CARTESIAN_POINT('Origin',(0.0332218842499744,0.,-0.815323436684413));
#11876=CARTESIAN_POINT('',(0.0663886785289726,1.,-0.813294868644317));
#11877=CARTESIAN_POINT('',(0.0663886785289726,0.,-0.813294868644317));
#11878=CARTESIAN_POINT('',(0.0332218842499744,1.,-0.815323436684413));
#11879=CARTESIAN_POINT('Origin',(0.0663886785289726,0.,-0.813294868644317));
#11880=CARTESIAN_POINT('',(0.0994453842186005,1.,-0.809917659739319));
#11881=CARTESIAN_POINT('',(0.0994453842186005,0.,-0.809917659739319));
#11882=CARTESIAN_POINT('',(0.0663886785289726,1.,-0.813294868644317));
#11883=CARTESIAN_POINT('Origin',(2.22044604925031E-16,-1.,-1.07625882986966));
#11884=CARTESIAN_POINT('',(0.163621780455751,-1.,-1.33259246319364));
#11885=CARTESIAN_POINT('',(0.0994453842186005,-1.,-0.809917659739319));
#11886=CARTESIAN_POINT('',(0.0994453842186005,-1.,-0.809917659739319));
#11887=CARTESIAN_POINT('',(0.0663886785289726,-1.,-0.813294868644317));
#11888=CARTESIAN_POINT('',(0.0663886785289726,-1.,-0.813294868644317));
#11889=CARTESIAN_POINT('',(0.0332218842499744,-1.,-0.815323436684413));
#11890=CARTESIAN_POINT('',(0.0332218842499744,-1.,-0.815323436684413));
#11891=CARTESIAN_POINT('',(2.22044604925031E-16,-1.,-0.816));
#11892=CARTESIAN_POINT('',(2.22044604925031E-16,-1.,-0.816));
#11893=CARTESIAN_POINT('',(-0.033221884249974,-1.,-0.815323436684413));
#11894=CARTESIAN_POINT('',(-0.033221884249974,-1.,-0.815323436684413));
#11895=CARTESIAN_POINT('',(-0.0663886785289722,-1.,-0.813294868644317));
#11896=CARTESIAN_POINT('',(-0.109232156609066,-1.,-1.33814913068855));
#11897=CARTESIAN_POINT('',(-0.109232156609066,-1.,-1.33814913068855));
#11898=CARTESIAN_POINT('',(-0.0546613992573715,-1.,-1.34148682119178));
#11899=CARTESIAN_POINT('',(-0.0546613992573715,-1.,-1.34148682119178));
#11900=CARTESIAN_POINT('',(2.22044604925031E-16,-1.,-1.3426));
#11901=CARTESIAN_POINT('',(2.22044604925031E-16,-1.,-1.3426));
#11902=CARTESIAN_POINT('',(0.054661399257372,-1.,-1.34148682119178));
#11903=CARTESIAN_POINT('',(0.054661399257372,-1.,-1.34148682119178));
#11904=CARTESIAN_POINT('',(0.109232156609067,-1.,-1.33814913068855));
#11905=CARTESIAN_POINT('',(0.109232156609067,-1.,-1.33814913068855));
#11906=CARTESIAN_POINT('',(0.163621780455751,-1.,-1.33259246319364));
#11907=CARTESIAN_POINT('Origin',(0.0663886785289726,0.,-0.813294868644317));
#11908=CARTESIAN_POINT('',(0.0663886785289726,0.,-0.813294868644317));
#11909=CARTESIAN_POINT('',(0.0994453842186005,0.,-0.809917659739319));
#11910=CARTESIAN_POINT('Origin',(0.0332218842499744,0.,-0.815323436684413));
#11911=CARTESIAN_POINT('',(0.0332218842499744,0.,-0.815323436684413));
#11912=CARTESIAN_POINT('Origin',(2.22044604925031E-16,0.,-0.816));
#11913=CARTESIAN_POINT('',(2.22044604925031E-16,0.,-0.816));
#11914=CARTESIAN_POINT('Origin',(-0.033221884249974,0.,-0.815323436684413));
#11915=CARTESIAN_POINT('',(-0.033221884249974,0.,-0.815323436684413));
#11916=CARTESIAN_POINT('Origin',(-0.0663886785289722,0.,-0.813294868644317));
#11917=CARTESIAN_POINT('Origin',(-0.109232156609066,0.,-1.33814913068855));
#11918=CARTESIAN_POINT('',(-0.109232156609066,1.,-1.33814913068855));
#11919=CARTESIAN_POINT('',(-0.109232156609066,1.,-1.33814913068855));
#11920=CARTESIAN_POINT('',(-0.109232156609066,0.,-1.33814913068855));
#11921=CARTESIAN_POINT('Origin',(-0.0546613992573715,0.,-1.34148682119178));
#11922=CARTESIAN_POINT('',(-0.0546613992573715,1.,-1.34148682119178));
#11923=CARTESIAN_POINT('',(-0.0546613992573715,1.,-1.34148682119178));
#11924=CARTESIAN_POINT('',(-0.0546613992573715,0.,-1.34148682119178));
#11925=CARTESIAN_POINT('Origin',(2.22044604925031E-16,0.,-1.3426));
#11926=CARTESIAN_POINT('',(2.22044604925031E-16,1.,-1.3426));
#11927=CARTESIAN_POINT('',(2.22044604925031E-16,1.,-1.3426));
#11928=CARTESIAN_POINT('',(2.22044604925031E-16,0.,-1.3426));
#11929=CARTESIAN_POINT('Origin',(0.054661399257372,0.,-1.34148682119178));
#11930=CARTESIAN_POINT('',(0.054661399257372,1.,-1.34148682119178));
#11931=CARTESIAN_POINT('',(0.054661399257372,1.,-1.34148682119178));
#11932=CARTESIAN_POINT('',(0.054661399257372,0.,-1.34148682119178));
#11933=CARTESIAN_POINT('Origin',(0.109232156609067,0.,-1.33814913068855));
#11934=CARTESIAN_POINT('',(0.109232156609067,1.,-1.33814913068855));
#11935=CARTESIAN_POINT('',(0.109232156609067,1.,-1.33814913068855));
#11936=CARTESIAN_POINT('',(0.109232156609067,0.,-1.33814913068855));
#11937=CARTESIAN_POINT('Origin',(0.163621780455751,0.,-1.33259246319364));
#11938=CARTESIAN_POINT('',(0.163621780455751,1.,-1.33259246319364));
#11939=CARTESIAN_POINT('',(0.163621780455751,1.,-1.33259246319364));
#11940=CARTESIAN_POINT('',(0.163621780455751,0.,-1.33259246319364));
#11941=CARTESIAN_POINT('Origin',(0.0994453842186005,0.,-0.809917659739319));
#11942=CARTESIAN_POINT('',(0.0994453842186005,1.,-0.809917659739319));
#11943=CARTESIAN_POINT('Origin',(2.22044604925031E-16,1.,-1.07625882986966));
#11944=CARTESIAN_POINT('Origin',(1.0722480357895,0.,-0.80799685008394));
#11945=CARTESIAN_POINT('',(0.651686576198591,1.,-0.491081058892071));
#11946=CARTESIAN_POINT('',(0.651686576198591,0.,-0.491081058892071));
#11947=CARTESIAN_POINT('',(1.0722480357895,1.,-0.80799685008394));
#11948=CARTESIAN_POINT('',(1.0722480357895,1.,-0.80799685008394));
#11949=CARTESIAN_POINT('',(1.0722480357895,-1.,-0.80799685008394));
#11950=CARTESIAN_POINT('',(1.0722480357895,0.,-0.80799685008394));
#11951=CARTESIAN_POINT('',(0.651686576198591,-1.,-0.491081058892071));
#11952=CARTESIAN_POINT('',(1.0722480357895,-1.,-0.80799685008394));
#11953=CARTESIAN_POINT('',(0.651686576198591,0.,-0.491081058892071));
#11954=CARTESIAN_POINT('Origin',(0.651686576198591,0.,-0.491081058892071));
#11955=CARTESIAN_POINT('',(0.67113967774902,1.,-0.464141716451927));
#11956=CARTESIAN_POINT('',(0.67113967774902,0.,-0.464141716451927));
#11957=CARTESIAN_POINT('',(0.651686576198591,1.,-0.491081058892071));
#11958=CARTESIAN_POINT('Origin',(0.651686576198591,0.,-0.491081058892071));
#11959=CARTESIAN_POINT('',(0.67113967774902,-1.,-0.464141716451927));
#11960=CARTESIAN_POINT('',(0.651686576198591,-1.,-0.491081058892071));
#11961=CARTESIAN_POINT('',(0.67113967774902,0.,-0.464141716451927));
#11962=CARTESIAN_POINT('Origin',(0.67113967774902,0.,-0.464141716451927));
#11963=CARTESIAN_POINT('',(0.689479866344548,1.,-0.43643271406427));
#11964=CARTESIAN_POINT('',(0.689479866344548,0.,-0.43643271406427));
#11965=CARTESIAN_POINT('',(0.67113967774902,1.,-0.464141716451927));
#11966=CARTESIAN_POINT('Origin',(0.689479866344548,0.,-0.43643271406427));
#11967=CARTESIAN_POINT('',(0.706676729488102,1.,-0.408));
#11968=CARTESIAN_POINT('',(0.706676729488102,0.,-0.408));
#11969=CARTESIAN_POINT('',(0.689479866344548,1.,-0.43643271406427));
#11970=CARTESIAN_POINT('Origin',(0.706676729488102,0.,-0.408));
#11971=CARTESIAN_POINT('',(0.722701750594522,1.,-0.378890722620142));
#11972=CARTESIAN_POINT('',(0.722701750594522,0.,-0.378890722620142));
#11973=CARTESIAN_POINT('',(0.706676729488102,1.,-0.408));
#11974=CARTESIAN_POINT('Origin',(0.722701750594522,0.,-0.378890722620142));
#11975=CARTESIAN_POINT('',(0.737528356277993,1.,-0.34915315219239));
#11976=CARTESIAN_POINT('',(0.737528356277993,0.,-0.34915315219239));
#11977=CARTESIAN_POINT('',(0.722701750594522,1.,-0.378890722620142));
#11978=CARTESIAN_POINT('Origin',(0.737528356277993,0.,-0.34915315219239));
#11979=CARTESIAN_POINT('',(0.751131960417191,1.,-0.318836600847247));
#11980=CARTESIAN_POINT('',(0.751131960417191,0.,-0.318836600847247));
#11981=CARTESIAN_POINT('',(0.737528356277993,1.,-0.34915315219239));
#11982=CARTESIAN_POINT('Origin',(0.932067487714439,-1.,-0.53812941493483));
#11983=CARTESIAN_POINT('',(1.23586981624525,-1.,-0.524595613109699));
#11984=CARTESIAN_POINT('',(0.751131960417191,-1.,-0.318836600847247));
#11985=CARTESIAN_POINT('',(0.751131960417191,-1.,-0.318836600847247));
#11986=CARTESIAN_POINT('',(0.737528356277993,-1.,-0.34915315219239));
#11987=CARTESIAN_POINT('',(0.737528356277993,-1.,-0.34915315219239));
#11988=CARTESIAN_POINT('',(0.722701750594522,-1.,-0.378890722620142));
#11989=CARTESIAN_POINT('',(0.722701750594522,-1.,-0.378890722620142));
#11990=CARTESIAN_POINT('',(0.706676729488102,-1.,-0.408));
#11991=CARTESIAN_POINT('',(0.706676729488102,-1.,-0.408));
#11992=CARTESIAN_POINT('',(0.689479866344548,-1.,-0.43643271406427));
#11993=CARTESIAN_POINT('',(0.689479866344548,-1.,-0.43643271406427));
#11994=CARTESIAN_POINT('',(0.67113967774902,-1.,-0.464141716451927));
#11995=CARTESIAN_POINT('',(1.10425506292382,-1.,-0.763672387877889));
#11996=CARTESIAN_POINT('',(1.10425506292382,-1.,-0.763672387877889));
#11997=CARTESIAN_POINT('',(1.13443096636543,-1.,-0.718081570959178));
#11998=CARTESIAN_POINT('',(1.13443096636543,-1.,-0.718081570959177));
#11999=CARTESIAN_POINT('',(1.16272570712099,-1.,-0.6713));
#12000=CARTESIAN_POINT('',(1.16272570712099,-1.,-0.6713));
#12001=CARTESIAN_POINT('',(1.1890923656228,-1.,-0.623405250232602));
#12002=CARTESIAN_POINT('',(1.1890923656228,-1.,-0.623405250232602));
#12003=CARTESIAN_POINT('',(1.21348721953288,-1.,-0.574476742810665));
#12004=CARTESIAN_POINT('',(1.21348721953288,-1.,-0.574476742810665));
#12005=CARTESIAN_POINT('',(1.23586981624525,-1.,-0.524595613109699));
#12006=CARTESIAN_POINT('Origin',(0.737528356277993,0.,-0.34915315219239));
#12007=CARTESIAN_POINT('',(0.737528356277993,0.,-0.34915315219239));
#12008=CARTESIAN_POINT('',(0.751131960417191,0.,-0.318836600847247));
#12009=CARTESIAN_POINT('Origin',(0.722701750594522,0.,-0.378890722620142));
#12010=CARTESIAN_POINT('',(0.722701750594522,0.,-0.378890722620142));
#12011=CARTESIAN_POINT('Origin',(0.706676729488102,0.,-0.408));
#12012=CARTESIAN_POINT('',(0.706676729488102,0.,-0.408));
#12013=CARTESIAN_POINT('Origin',(0.689479866344548,0.,-0.43643271406427));
#12014=CARTESIAN_POINT('',(0.689479866344548,0.,-0.43643271406427));
#12015=CARTESIAN_POINT('Origin',(0.67113967774902,0.,-0.464141716451927));
#12016=CARTESIAN_POINT('Origin',(1.10425506292382,0.,-0.763672387877889));
#12017=CARTESIAN_POINT('',(1.10425506292382,1.,-0.763672387877889));
#12018=CARTESIAN_POINT('',(1.10425506292382,1.,-0.763672387877889));
#12019=CARTESIAN_POINT('',(1.10425506292382,0.,-0.763672387877889));
#12020=CARTESIAN_POINT('Origin',(1.13443096636543,0.,-0.718081570959177));
#12021=CARTESIAN_POINT('',(1.13443096636543,1.,-0.718081570959178));
#12022=CARTESIAN_POINT('',(1.13443096636543,1.,-0.718081570959177));
#12023=CARTESIAN_POINT('',(1.13443096636543,0.,-0.718081570959177));
#12024=CARTESIAN_POINT('Origin',(1.16272570712099,0.,-0.6713));
#12025=CARTESIAN_POINT('',(1.16272570712099,1.,-0.6713));
#12026=CARTESIAN_POINT('',(1.16272570712099,1.,-0.6713));
#12027=CARTESIAN_POINT('',(1.16272570712099,0.,-0.6713));
#12028=CARTESIAN_POINT('Origin',(1.1890923656228,0.,-0.623405250232602));
#12029=CARTESIAN_POINT('',(1.1890923656228,1.,-0.623405250232602));
#12030=CARTESIAN_POINT('',(1.1890923656228,1.,-0.623405250232602));
#12031=CARTESIAN_POINT('',(1.1890923656228,0.,-0.623405250232602));
#12032=CARTESIAN_POINT('Origin',(1.21348721953288,0.,-0.574476742810665));
#12033=CARTESIAN_POINT('',(1.21348721953288,1.,-0.574476742810665));
#12034=CARTESIAN_POINT('',(1.21348721953288,1.,-0.574476742810665));
#12035=CARTESIAN_POINT('',(1.21348721953288,0.,-0.574476742810665));
#12036=CARTESIAN_POINT('Origin',(1.23586981624525,0.,-0.524595613109699));
#12037=CARTESIAN_POINT('',(1.23586981624525,1.,-0.524595613109699));
#12038=CARTESIAN_POINT('',(1.23586981624525,1.,-0.524595613109699));
#12039=CARTESIAN_POINT('',(1.23586981624525,0.,-0.524595613109699));
#12040=CARTESIAN_POINT('Origin',(0.751131960417191,0.,-0.318836600847247));
#12041=CARTESIAN_POINT('',(0.751131960417191,1.,-0.318836600847247));
#12042=CARTESIAN_POINT('Origin',(0.932067487714439,1.,-0.53812941493483));
#12043=CARTESIAN_POINT('Origin',(-1.23586981624525,0.,-0.524595613109699));
#12044=CARTESIAN_POINT('',(-0.751131960417191,1.,-0.318836600847248));
#12045=CARTESIAN_POINT('',(-0.751131960417191,0.,-0.318836600847248));
#12046=CARTESIAN_POINT('',(-1.23586981624525,1.,-0.524595613109699));
#12047=CARTESIAN_POINT('',(-1.23586981624525,1.,-0.524595613109699));
#12048=CARTESIAN_POINT('',(-1.23586981624525,-1.,-0.524595613109699));
#12049=CARTESIAN_POINT('',(-1.23586981624525,0.,-0.524595613109699));
#12050=CARTESIAN_POINT('',(-0.751131960417191,-1.,-0.318836600847248));
#12051=CARTESIAN_POINT('',(-1.23586981624525,-1.,-0.524595613109699));
#12052=CARTESIAN_POINT('',(-0.751131960417191,0.,-0.318836600847248));
#12053=CARTESIAN_POINT('Origin',(-0.751131960417191,0.,-0.318836600847248));
#12054=CARTESIAN_POINT('',(-0.737528356277993,1.,-0.34915315219239));
#12055=CARTESIAN_POINT('',(-0.737528356277993,0.,-0.34915315219239));
#12056=CARTESIAN_POINT('',(-0.751131960417191,1.,-0.318836600847248));
#12057=CARTESIAN_POINT('Origin',(-0.751131960417191,0.,-0.318836600847248));
#12058=CARTESIAN_POINT('',(-0.737528356277993,-1.,-0.34915315219239));
#12059=CARTESIAN_POINT('',(-0.751131960417191,-1.,-0.318836600847248));
#12060=CARTESIAN_POINT('',(-0.737528356277993,0.,-0.34915315219239));
#12061=CARTESIAN_POINT('Origin',(-0.737528356277993,0.,-0.34915315219239));
#12062=CARTESIAN_POINT('',(-0.722701750594522,1.,-0.378890722620143));
#12063=CARTESIAN_POINT('',(-0.722701750594522,0.,-0.378890722620143));
#12064=CARTESIAN_POINT('',(-0.737528356277993,1.,-0.34915315219239));
#12065=CARTESIAN_POINT('Origin',(-0.722701750594522,0.,-0.378890722620143));
#12066=CARTESIAN_POINT('',(-0.706676729488102,1.,-0.408));
#12067=CARTESIAN_POINT('',(-0.706676729488102,0.,-0.408));
#12068=CARTESIAN_POINT('',(-0.722701750594522,1.,-0.378890722620143));
#12069=CARTESIAN_POINT('Origin',(-0.706676729488102,0.,-0.408));
#12070=CARTESIAN_POINT('',(-0.689479866344548,1.,-0.43643271406427));
#12071=CARTESIAN_POINT('',(-0.689479866344548,0.,-0.43643271406427));
#12072=CARTESIAN_POINT('',(-0.706676729488102,1.,-0.408));
#12073=CARTESIAN_POINT('Origin',(-0.689479866344548,0.,-0.43643271406427));
#12074=CARTESIAN_POINT('',(-0.67113967774902,1.,-0.464141716451927));
#12075=CARTESIAN_POINT('',(-0.67113967774902,0.,-0.464141716451927));
#12076=CARTESIAN_POINT('',(-0.689479866344548,1.,-0.43643271406427));
#12077=CARTESIAN_POINT('Origin',(-0.67113967774902,0.,-0.464141716451927));
#12078=CARTESIAN_POINT('',(-0.651686576198591,1.,-0.491081058892072));
#12079=CARTESIAN_POINT('',(-0.651686576198591,0.,-0.491081058892072));
#12080=CARTESIAN_POINT('',(-0.67113967774902,1.,-0.464141716451927));
#12081=CARTESIAN_POINT('Origin',(-0.932067487714439,-1.,-0.53812941493483));
#12082=CARTESIAN_POINT('',(-1.0722480357895,-1.,-0.80799685008394));
#12083=CARTESIAN_POINT('',(-0.651686576198591,-1.,-0.491081058892072));
#12084=CARTESIAN_POINT('',(-0.651686576198591,-1.,-0.491081058892072));
#12085=CARTESIAN_POINT('',(-0.67113967774902,-1.,-0.464141716451927));
#12086=CARTESIAN_POINT('',(-0.67113967774902,-1.,-0.464141716451927));
#12087=CARTESIAN_POINT('',(-0.689479866344548,-1.,-0.43643271406427));
#12088=CARTESIAN_POINT('',(-0.689479866344548,-1.,-0.43643271406427));
#12089=CARTESIAN_POINT('',(-0.706676729488102,-1.,-0.408));
#12090=CARTESIAN_POINT('',(-0.706676729488102,-1.,-0.408));
#12091=CARTESIAN_POINT('',(-0.722701750594522,-1.,-0.378890722620143));
#12092=CARTESIAN_POINT('',(-0.722701750594522,-1.,-0.378890722620143));
#12093=CARTESIAN_POINT('',(-0.737528356277993,-1.,-0.34915315219239));
#12094=CARTESIAN_POINT('',(-1.21348721953288,-1.,-0.574476742810665));
#12095=CARTESIAN_POINT('',(-1.21348721953288,-1.,-0.574476742810665));
#12096=CARTESIAN_POINT('',(-1.1890923656228,-1.,-0.623405250232602));
#12097=CARTESIAN_POINT('',(-1.1890923656228,-1.,-0.623405250232602));
#12098=CARTESIAN_POINT('',(-1.16272570712099,-1.,-0.6713));
#12099=CARTESIAN_POINT('',(-1.16272570712099,-1.,-0.6713));
#12100=CARTESIAN_POINT('',(-1.13443096636543,-1.,-0.718081570959178));
#12101=CARTESIAN_POINT('',(-1.13443096636543,-1.,-0.718081570959178));
#12102=CARTESIAN_POINT('',(-1.10425506292382,-1.,-0.763672387877889));
#12103=CARTESIAN_POINT('',(-1.10425506292382,-1.,-0.763672387877889));
#12104=CARTESIAN_POINT('',(-1.0722480357895,-1.,-0.80799685008394));
#12105=CARTESIAN_POINT('Origin',(-0.67113967774902,0.,-0.464141716451927));
#12106=CARTESIAN_POINT('',(-0.67113967774902,0.,-0.464141716451927));
#12107=CARTESIAN_POINT('',(-0.651686576198591,0.,-0.491081058892072));
#12108=CARTESIAN_POINT('Origin',(-0.689479866344548,0.,-0.43643271406427));
#12109=CARTESIAN_POINT('',(-0.689479866344548,0.,-0.43643271406427));
#12110=CARTESIAN_POINT('Origin',(-0.706676729488102,0.,-0.408));
#12111=CARTESIAN_POINT('',(-0.706676729488102,0.,-0.408));
#12112=CARTESIAN_POINT('Origin',(-0.722701750594522,0.,-0.378890722620143));
#12113=CARTESIAN_POINT('',(-0.722701750594522,0.,-0.378890722620143));
#12114=CARTESIAN_POINT('Origin',(-0.737528356277993,0.,-0.34915315219239));
#12115=CARTESIAN_POINT('Origin',(-1.21348721953288,0.,-0.574476742810665));
#12116=CARTESIAN_POINT('',(-1.21348721953288,1.,-0.574476742810665));
#12117=CARTESIAN_POINT('',(-1.21348721953288,1.,-0.574476742810665));
#12118=CARTESIAN_POINT('',(-1.21348721953288,0.,-0.574476742810665));
#12119=CARTESIAN_POINT('Origin',(-1.1890923656228,0.,-0.623405250232602));
#12120=CARTESIAN_POINT('',(-1.1890923656228,1.,-0.623405250232602));
#12121=CARTESIAN_POINT('',(-1.1890923656228,1.,-0.623405250232602));
#12122=CARTESIAN_POINT('',(-1.1890923656228,0.,-0.623405250232602));
#12123=CARTESIAN_POINT('Origin',(-1.16272570712099,0.,-0.6713));
#12124=CARTESIAN_POINT('',(-1.16272570712099,1.,-0.6713));
#12125=CARTESIAN_POINT('',(-1.16272570712099,1.,-0.6713));
#12126=CARTESIAN_POINT('',(-1.16272570712099,0.,-0.6713));
#12127=CARTESIAN_POINT('Origin',(-1.13443096636543,0.,-0.718081570959178));
#12128=CARTESIAN_POINT('',(-1.13443096636543,1.,-0.718081570959178));
#12129=CARTESIAN_POINT('',(-1.13443096636543,1.,-0.718081570959178));
#12130=CARTESIAN_POINT('',(-1.13443096636543,0.,-0.718081570959178));
#12131=CARTESIAN_POINT('Origin',(-1.10425506292382,0.,-0.763672387877889));
#12132=CARTESIAN_POINT('',(-1.10425506292382,1.,-0.763672387877889));
#12133=CARTESIAN_POINT('',(-1.10425506292382,1.,-0.763672387877889));
#12134=CARTESIAN_POINT('',(-1.10425506292382,0.,-0.763672387877889));
#12135=CARTESIAN_POINT('Origin',(-1.0722480357895,0.,-0.80799685008394));
#12136=CARTESIAN_POINT('',(-1.0722480357895,1.,-0.80799685008394));
#12137=CARTESIAN_POINT('',(-1.0722480357895,1.,-0.80799685008394));
#12138=CARTESIAN_POINT('',(-1.0722480357895,0.,-0.80799685008394));
#12139=CARTESIAN_POINT('Origin',(-0.651686576198591,0.,-0.491081058892072));
#12140=CARTESIAN_POINT('',(-0.651686576198591,1.,-0.491081058892072));
#12141=CARTESIAN_POINT('Origin',(-0.932067487714439,1.,-0.53812941493483));
#12142=CARTESIAN_POINT('Origin',(0.16362178045575,0.,1.33259246319364));
#12143=CARTESIAN_POINT('',(0.0994453842185998,1.,0.809917659739319));
#12144=CARTESIAN_POINT('',(0.0994453842185998,0.,0.809917659739319));
#12145=CARTESIAN_POINT('',(0.16362178045575,1.,1.33259246319364));
#12146=CARTESIAN_POINT('',(0.16362178045575,1.,1.33259246319364));
#12147=CARTESIAN_POINT('',(0.16362178045575,-1.,1.33259246319364));
#12148=CARTESIAN_POINT('',(0.16362178045575,0.,1.33259246319364));
#12149=CARTESIAN_POINT('',(0.0994453842185998,-1.,0.809917659739319));
#12150=CARTESIAN_POINT('',(0.16362178045575,-1.,1.33259246319364));
#12151=CARTESIAN_POINT('',(0.0994453842185998,0.,0.809917659739319));
#12152=CARTESIAN_POINT('Origin',(0.0994453842185998,0.,0.809917659739319));
#12153=CARTESIAN_POINT('',(0.0663886785289718,1.,0.813294868644317));
#12154=CARTESIAN_POINT('',(0.0663886785289718,0.,0.813294868644317));
#12155=CARTESIAN_POINT('',(0.0994453842185998,1.,0.809917659739319));
#12156=CARTESIAN_POINT('Origin',(0.0994453842185998,0.,0.809917659739319));
#12157=CARTESIAN_POINT('',(0.0663886785289718,-1.,0.813294868644317));
#12158=CARTESIAN_POINT('',(0.0994453842185998,-1.,0.809917659739319));
#12159=CARTESIAN_POINT('',(0.0663886785289718,0.,0.813294868644317));
#12160=CARTESIAN_POINT('Origin',(0.0663886785289718,0.,0.813294868644317));
#12161=CARTESIAN_POINT('',(0.0332218842499737,1.,0.815323436684413));
#12162=CARTESIAN_POINT('',(0.0332218842499737,0.,0.815323436684413));
#12163=CARTESIAN_POINT('',(0.0663886785289718,1.,0.813294868644317));
#12164=CARTESIAN_POINT('Origin',(0.0332218842499737,0.,0.815323436684413));
#12165=CARTESIAN_POINT('',(-4.9960036108132E-16,1.,0.816));
#12166=CARTESIAN_POINT('',(-4.9960036108132E-16,0.,0.816));
#12167=CARTESIAN_POINT('',(0.0332218842499737,1.,0.815323436684413));
#12168=CARTESIAN_POINT('Origin',(-4.9960036108132E-16,0.,0.816));
#12169=CARTESIAN_POINT('',(-0.0332218842499747,1.,0.815323436684413));
#12170=CARTESIAN_POINT('',(-0.0332218842499747,0.,0.815323436684413));
#12171=CARTESIAN_POINT('',(-4.9960036108132E-16,1.,0.816));
#12172=CARTESIAN_POINT('Origin',(-0.0332218842499747,0.,0.815323436684413));
#12173=CARTESIAN_POINT('',(-0.0663886785289729,1.,0.813294868644317));
#12174=CARTESIAN_POINT('',(-0.0663886785289729,0.,0.813294868644317));
#12175=CARTESIAN_POINT('',(-0.0332218842499747,1.,0.815323436684413));
#12176=CARTESIAN_POINT('Origin',(-0.0663886785289729,0.,0.813294868644317));
#12177=CARTESIAN_POINT('',(-0.0994453842186008,1.,0.809917659739319));
#12178=CARTESIAN_POINT('',(-0.0994453842186008,0.,0.809917659739319));
#12179=CARTESIAN_POINT('',(-0.0663886785289729,1.,0.813294868644317));
#12180=CARTESIAN_POINT('Origin',(-6.10622663543836E-16,-1.,1.07625882986966));
#12181=CARTESIAN_POINT('',(-0.163621780455752,-1.,1.33259246319364));
#12182=CARTESIAN_POINT('',(-0.0994453842186008,-1.,0.809917659739319));
#12183=CARTESIAN_POINT('',(-0.0994453842186008,-1.,0.809917659739319));
#12184=CARTESIAN_POINT('',(-0.0663886785289729,-1.,0.813294868644317));
#12185=CARTESIAN_POINT('',(-0.0663886785289729,-1.,0.813294868644317));
#12186=CARTESIAN_POINT('',(-0.0332218842499747,-1.,0.815323436684413));
#12187=CARTESIAN_POINT('',(-0.0332218842499747,-1.,0.815323436684413));
#12188=CARTESIAN_POINT('',(-4.9960036108132E-16,-1.,0.816));
#12189=CARTESIAN_POINT('',(-4.9960036108132E-16,-1.,0.816));
#12190=CARTESIAN_POINT('',(0.0332218842499737,-1.,0.815323436684413));
#12191=CARTESIAN_POINT('',(0.0332218842499737,-1.,0.815323436684413));
#12192=CARTESIAN_POINT('',(0.0663886785289718,-1.,0.813294868644317));
#12193=CARTESIAN_POINT('',(0.109232156609066,-1.,1.33814913068855));
#12194=CARTESIAN_POINT('',(0.109232156609066,-1.,1.33814913068855));
#12195=CARTESIAN_POINT('',(0.054661399257371,-1.,1.34148682119178));
#12196=CARTESIAN_POINT('',(0.054661399257371,-1.,1.34148682119178));
#12197=CARTESIAN_POINT('',(-7.7715611723761E-16,-1.,1.3426));
#12198=CARTESIAN_POINT('',(-7.7715611723761E-16,-1.,1.3426));
#12199=CARTESIAN_POINT('',(-0.0546613992573726,-1.,1.34148682119178));
#12200=CARTESIAN_POINT('',(-0.0546613992573726,-1.,1.34148682119178));
#12201=CARTESIAN_POINT('',(-0.109232156609067,-1.,1.33814913068855));
#12202=CARTESIAN_POINT('',(-0.109232156609067,-1.,1.33814913068855));
#12203=CARTESIAN_POINT('',(-0.163621780455752,-1.,1.33259246319364));
#12204=CARTESIAN_POINT('Origin',(-0.0663886785289729,0.,0.813294868644317));
#12205=CARTESIAN_POINT('',(-0.0663886785289729,0.,0.813294868644317));
#12206=CARTESIAN_POINT('',(-0.0994453842186008,0.,0.809917659739319));
#12207=CARTESIAN_POINT('Origin',(-0.0332218842499747,0.,0.815323436684413));
#12208=CARTESIAN_POINT('',(-0.0332218842499747,0.,0.815323436684413));
#12209=CARTESIAN_POINT('Origin',(-4.9960036108132E-16,0.,0.816));
#12210=CARTESIAN_POINT('',(-4.9960036108132E-16,0.,0.816));
#12211=CARTESIAN_POINT('Origin',(0.0332218842499737,0.,0.815323436684413));
#12212=CARTESIAN_POINT('',(0.0332218842499737,0.,0.815323436684413));
#12213=CARTESIAN_POINT('Origin',(0.0663886785289718,0.,0.813294868644317));
#12214=CARTESIAN_POINT('Origin',(0.109232156609066,0.,1.33814913068855));
#12215=CARTESIAN_POINT('',(0.109232156609066,1.,1.33814913068855));
#12216=CARTESIAN_POINT('',(0.109232156609066,1.,1.33814913068855));
#12217=CARTESIAN_POINT('',(0.109232156609066,0.,1.33814913068855));
#12218=CARTESIAN_POINT('Origin',(0.054661399257371,0.,1.34148682119178));
#12219=CARTESIAN_POINT('',(0.054661399257371,1.,1.34148682119178));
#12220=CARTESIAN_POINT('',(0.054661399257371,1.,1.34148682119178));
#12221=CARTESIAN_POINT('',(0.054661399257371,0.,1.34148682119178));
#12222=CARTESIAN_POINT('Origin',(-7.7715611723761E-16,0.,1.3426));
#12223=CARTESIAN_POINT('',(-7.7715611723761E-16,1.,1.3426));
#12224=CARTESIAN_POINT('',(-7.7715611723761E-16,1.,1.3426));
#12225=CARTESIAN_POINT('',(-7.7715611723761E-16,0.,1.3426));
#12226=CARTESIAN_POINT('Origin',(-0.0546613992573726,0.,1.34148682119178));
#12227=CARTESIAN_POINT('',(-0.0546613992573726,1.,1.34148682119178));
#12228=CARTESIAN_POINT('',(-0.0546613992573726,1.,1.34148682119178));
#12229=CARTESIAN_POINT('',(-0.0546613992573726,0.,1.34148682119178));
#12230=CARTESIAN_POINT('Origin',(-0.109232156609067,0.,1.33814913068855));
#12231=CARTESIAN_POINT('',(-0.109232156609067,1.,1.33814913068855));
#12232=CARTESIAN_POINT('',(-0.109232156609067,1.,1.33814913068855));
#12233=CARTESIAN_POINT('',(-0.109232156609067,0.,1.33814913068855));
#12234=CARTESIAN_POINT('Origin',(-0.163621780455752,0.,1.33259246319364));
#12235=CARTESIAN_POINT('',(-0.163621780455752,1.,1.33259246319364));
#12236=CARTESIAN_POINT('',(-0.163621780455752,1.,1.33259246319364));
#12237=CARTESIAN_POINT('',(-0.163621780455752,0.,1.33259246319364));
#12238=CARTESIAN_POINT('Origin',(-0.0994453842186008,0.,0.809917659739319));
#12239=CARTESIAN_POINT('',(-0.0994453842186008,1.,0.809917659739319));
#12240=CARTESIAN_POINT('Origin',(-6.10622663543836E-16,1.,1.07625882986966));
#12327=UNCERTAINTY_MEASURE_WITH_UNIT(LENGTH_MEASURE(0.001),#12344,
'DISTANCE_ACCURACY_VALUE',
'Maximum model space distance between geometric entities at asserted c
onnectivities');
#12329=UNCERTAINTY_MEASURE_WITH_UNIT(LENGTH_MEASURE(0.001),#12344,
'DISTANCE_ACCURACY_VALUE',
'Maximum model space distance between geometric entities at asserted c
onnectivities');
#12341=(
GEOMETRIC_REPRESENTATION_CONTEXT(3)
GLOBAL_UNCERTAINTY_ASSIGNED_CONTEXT((#12327))
GLOBAL_UNIT_ASSIGNED_CONTEXT((#12344,#12346,#12347))
REPRESENTATION_CONTEXT('','3D')
);
#12343=(
GEOMETRIC_REPRESENTATION_CONTEXT(3)
GLOBAL_UNCERTAINTY_ASSIGNED_CONTEXT((#12329))
GLOBAL_UNIT_ASSIGNED_CONTEXT((#12344,#12346,#12347))
REPRESENTATION_CONTEXT('','3D')
);
#12344=(
LENGTH_UNIT()
NAMED_UNIT(*)
SI_UNIT(.CENTI.,.METRE.)
);
#12346=(
NAMED_UNIT(*)
PLANE_ANGLE_UNIT()
SI_UNIT($,.RADIAN.)
);
#12347=(
NAMED_UNIT(*)
SI_UNIT($,.STERADIAN.)
SOLID_ANGLE_UNIT()
);
#12359=SHAPE_DEFINITION_REPRESENTATION(#12372,#12406);
#12372=PRODUCT_DEFINITION_SHAPE('',$,#12420);
#12406=SHAPE_REPRESENTATION('',(#7853),#12341);
#12408=PRODUCT_DEFINITION_CONTEXT('part definition',#12449,'design');
#12420=PRODUCT_DEFINITION('Spider','Spider',#12433,#12408);
#12433=PRODUCT_DEFINITION_FORMATION('',$,#12462);
#12449=APPLICATION_CONTEXT(
'Core Data for Automotive Mechanical Design Process');
#12450=PRODUCT_CONTEXT('part definition',#12449,'mechanical');
#12462=PRODUCT('Spider','Spider','Spider',(#12450));
#12520=COLOUR_RGB('Sky Blue',0.24,0.69,0.87);
#12521=FILL_AREA_STYLE_COLOUR('',#12520);
#12522=FILL_AREA_STYLE('',(#12521));
#12523=SURFACE_STYLE_FILL_AREA(#12522);
#12524=SURFACE_SIDE_STYLE('',(#12523));
#12525=SURFACE_STYLE_USAGE(.BOTH.,#12524);
#12526=PRESENTATION_STYLE_ASSIGNMENT((#12525));
ENDSEC;
END-ISO-10303-21;
